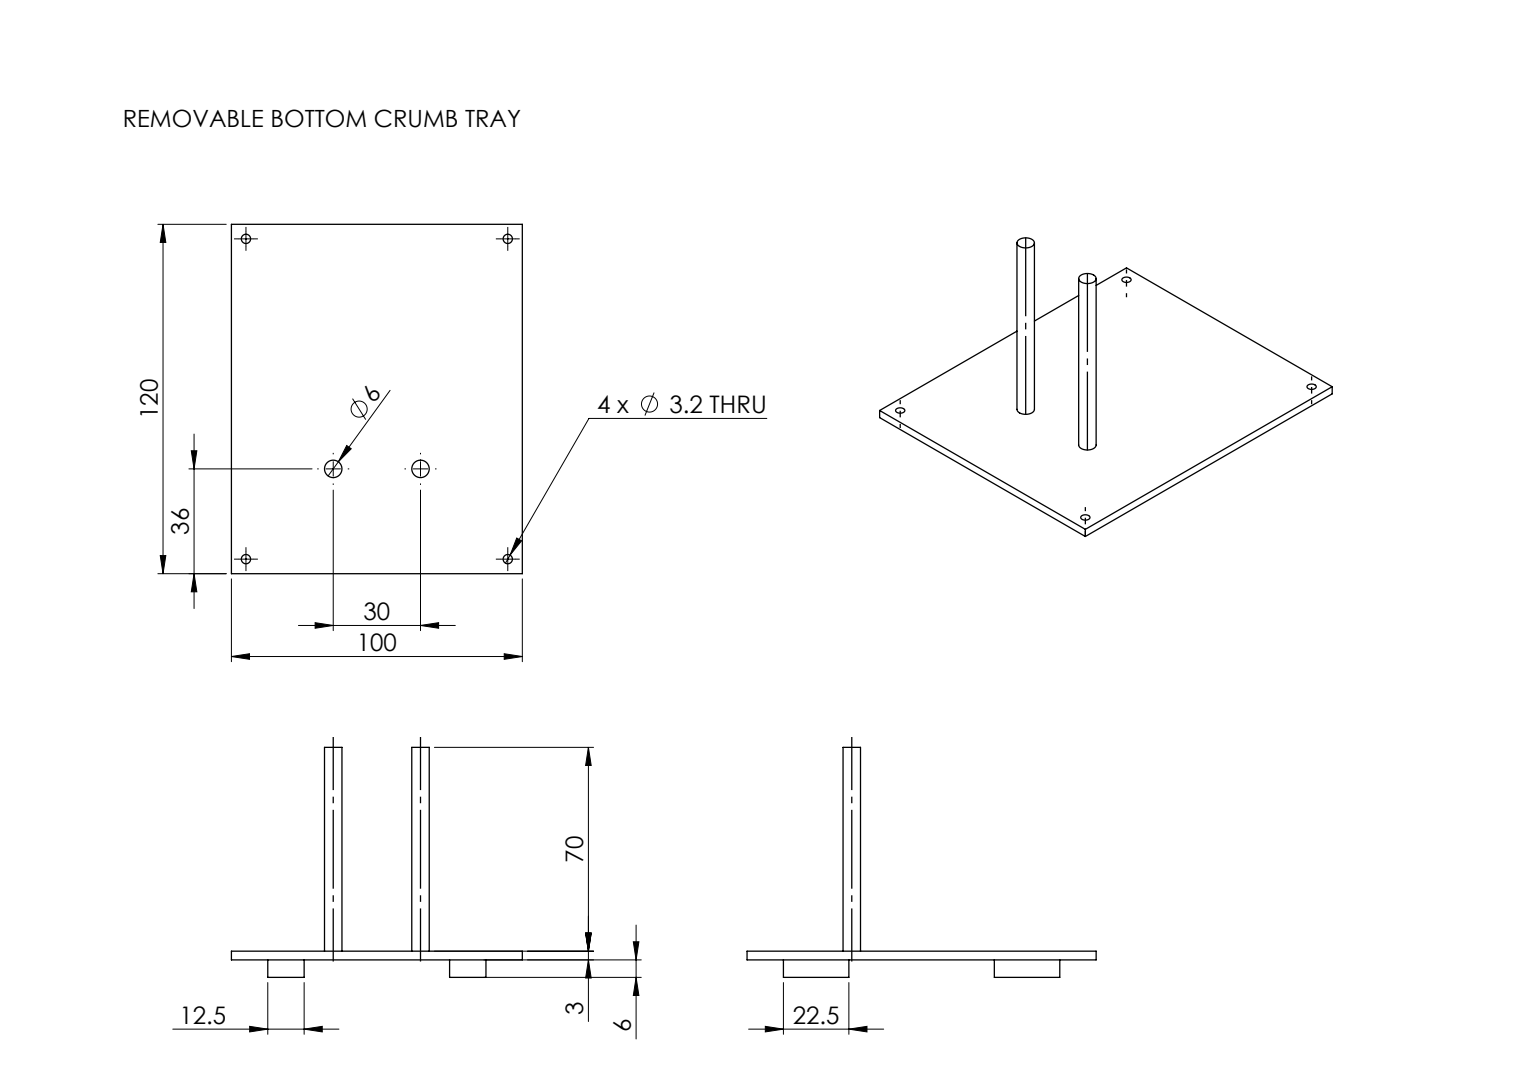
ISO-10303-21;
HEADER;
FILE_DESCRIPTION (('STEP AP214'),
    '1' );
FILE_NAME ('Removable Bottom Crumb Tray.step',
    '2026-10-08T14:41:38',
    ( '' ),
    ( '' ),
    'SwSTEP 2.0',
    'SolidWorks 2026',
    '' );
FILE_SCHEMA (( 'AUTOMOTIVE_DESIGN' ));
ENDSEC;

DATA;
#10=FACE_OUTER_BOUND ( 'NONE', #5278, .T. ) ;
#18=EDGE_CURVE ( 'NONE', #5079, #4517, #16249, .T. ) ;
#22=VECTOR ( 'NONE', #16690, 1000.000000000000000 ) ;
#26=EDGE_CURVE ( 'NONE', #14106, #19091, #11969, .T. ) ;
#36=EDGE_CURVE ( 'NONE', #18345, #7828, #11830, .T. ) ;
#43=CARTESIAN_POINT ( 'NONE',  ( 37.50000000000000711, -6.000000000000000000, -45.00000000000000000 ) ) ;
#62=CARTESIAN_POINT ( 'NONE',  ( -37.50000000000002132, 0.000000000000000000, 44.99999999999997868 ) ) ;
#75=FACE_OUTER_BOUND ( 'NONE', #12049, .T. ) ;
#86=LINE ( 'NONE', #12030, #9433 ) ;
#109=VERTEX_POINT ( 'NONE', #11046 ) ;
#116=CARTESIAN_POINT ( 'NONE',  ( -44.99999999999998579, 0.000000000000000000, -55.00000000000000000 ) ) ;
#124=EDGE_CURVE ( 'NONE', #10346, #18340, #3322, .T. ) ;
#138=EDGE_CURVE ( 'NONE', #19239, #1798, #9382, .T. ) ;
#157=DIRECTION ( 'NONE',  ( 1.000000000000000000, 0.000000000000000000, -7.709882115452476934E-17 ) ) ;
#163=LINE ( 'NONE', #1934, #7064 ) ;
#172=DIRECTION ( 'NONE',  ( -2.973811673103096679E-16, 0.000000000000000000, 1.000000000000000000 ) ) ;
#197=EDGE_LOOP ( 'NONE', ( #16436, #17465, #12376, #16579 ) ) ;
#223=LINE ( 'NONE', #13638, #15855 ) ;
#252=LINE ( 'NONE', #16158, #15418 ) ;
#255=DIRECTION ( 'NONE',  ( 0.000000000000000000, 0.000000000000000000, -1.000000000000000000 ) ) ;
#273=AXIS2_PLACEMENT_3D ( 'NONE', #16902, #3471, #9445 ) ;
#276=EDGE_CURVE ( 'NONE', #17921, #11844, #16850, .T. ) ;
#284=CARTESIAN_POINT ( 'NONE',  ( 14.99999999999998579, 3.000000000000000000, 26.99999999999997158 ) ) ;
#303=EDGE_CURVE ( 'NONE', #628, #8146, #5681, .T. ) ;
#315=LINE ( 'NONE', #7965, #7095 ) ;
#320=ORIENTED_EDGE ( 'NONE', *, *, #11499, .F. ) ;
#366=VECTOR ( 'NONE', #8391, 1000.000000000000000 ) ;
#370=LINE ( 'NONE', #15368, #6453 ) ;
#372=VECTOR ( 'NONE', #7310, 1000.000000000000000 ) ;
#378=ADVANCED_FACE ( 'NONE', ( #14562 ), #11224, .T. ) ;
#384=EDGE_CURVE ( 'NONE', #16449, #5562, #9851, .T. ) ;
#393=VECTOR ( 'NONE', #11200, 1000.000000000000000 ) ;
#394=EDGE_LOOP ( 'NONE', ( #6539, #4312, #7875, #13610 ) ) ;
#404=ORIENTED_EDGE ( 'NONE', *, *, #14193, .T. ) ;
#407=DIRECTION ( 'NONE',  ( -0.000000000000000000, -1.000000000000000000, -0.000000000000000000 ) ) ;
#423=EDGE_CURVE ( 'NONE', #13623, #11742, #14277, .T. ) ;
#428=VERTEX_POINT ( 'NONE', #16040 ) ;
#479=DIRECTION ( 'NONE',  ( -0.000000000000000000, -1.000000000000000000, -0.000000000000000000 ) ) ;
#497=DIRECTION ( 'NONE',  ( -1.000000000000000000, 0.000000000000000000, -9.251858538542970348E-17 ) ) ;
#510=EDGE_CURVE ( 'NONE', #15185, #7828, #9171, .T. ) ;
#526=EDGE_CURVE ( 'NONE', #18598, #13355, #19142, .T. ) ;
#528=EDGE_CURVE ( 'NONE', #3513, #14696, #14857, .T. ) ;
#539=DIRECTION ( 'NONE',  ( 0.000000000000000000, 0.000000000000000000, -1.000000000000000000 ) ) ;
#547=DIRECTION ( 'NONE',  ( 0.000000000000000000, 0.000000000000000000, -1.000000000000000000 ) ) ;
#553=ORIENTED_EDGE ( 'NONE', *, *, #12530, .T. ) ;
#561=EDGE_LOOP ( 'NONE', ( #1541, #12212 ) ) ;
#569=EDGE_CURVE ( 'NONE', #5562, #14997, #2796, .T. ) ;
#571=ADVANCED_BREP_SHAPE_REPRESENTATION ( '', ( #16938, #1791 ), #5851 ) ;
#572=DIRECTION ( 'NONE',  ( -1.541976423090495633E-16, 0.000000000000000000, 1.000000000000000000 ) ) ;
#577=ORIENTED_EDGE ( 'NONE', *, *, #17798, .T. ) ;
#589=EDGE_LOOP ( 'NONE', ( #3897, #9508, #16057, #4812 ) ) ;
#590=CARTESIAN_POINT ( 'NONE',  ( 44.99999999999998579, 0.000000000000000000, -54.99999999999998579 ) ) ;
#600=CARTESIAN_POINT ( 'NONE',  ( 44.99999999999998579, 3.000000000000000000, -53.39999999999999147 ) ) ;
#616=EDGE_CURVE ( 'NONE', #16789, #4517, #9072, .T. ) ;
#619=FACE_BOUND ( 'NONE', #18932, .T. ) ;
#628=VERTEX_POINT ( 'NONE', #13272 ) ;
#639=FACE_OUTER_BOUND ( 'NONE', #6765, .T. ) ;
#648=DIRECTION ( 'NONE',  ( -0.000000000000000000, -1.000000000000000000, -0.000000000000000000 ) ) ;
#654=EDGE_CURVE ( 'NONE', #10863, #8734, #2898, .T. ) ;
#673=PLANE ( 'NONE',  #15685 ) ;
#686=FACE_BOUND ( 'NONE', #17329, .T. ) ;
#717=VERTEX_POINT ( 'NONE', #15447 ) ;
#739=DIRECTION ( 'NONE',  ( 0.000000000000000000, -1.000000000000000000, 0.000000000000000000 ) ) ;
#762=EDGE_LOOP ( 'NONE', ( #16079, #7445, #9963, #6983 ) ) ;
#785=ADVANCED_FACE ( 'NONE', ( #639 ), #6236, .F. ) ;
#795=DIRECTION ( 'NONE',  ( -0.000000000000000000, -1.000000000000000000, -0.000000000000000000 ) ) ;
#821=EDGE_CURVE ( 'NONE', #5173, #12630, #4675, .T. ) ;
#830=CARTESIAN_POINT ( 'NONE',  ( -50.00000000000002132, 0.000000000000000000, -60.00000000000002132 ) ) ;
#848=EDGE_CURVE ( 'NONE', #5969, #14590, #7908, .T. ) ;
#865=ORIENTED_EDGE ( 'NONE', *, *, #15879, .F. ) ;
#887=EDGE_CURVE ( 'NONE', #16466, #19197, #4055, .T. ) ;
#894=DIRECTION ( 'NONE',  ( 0.000000000000000000, 0.000000000000000000, -1.000000000000000000 ) ) ;
#904=VECTOR ( 'NONE', #4505, 1000.000000000000000 ) ;
#945=AXIS2_PLACEMENT_3D ( 'NONE', #1086, #16280, #1182 ) ;
#985=CARTESIAN_POINT ( 'NONE',  ( -32.50000000000002132, -6.000000000000000000, -42.50000000000001421 ) ) ;
#1005=DIRECTION ( 'NONE',  ( -0.000000000000000000, -1.000000000000000000, -0.000000000000000000 ) ) ;
#1066=DIRECTION ( 'NONE',  ( 7.304098846218135653E-17, 0.000000000000000000, -1.000000000000000000 ) ) ;
#1069=DIRECTION ( 'NONE',  ( 0.000000000000000000, 0.000000000000000000, -1.000000000000000000 ) ) ;
#1086=CARTESIAN_POINT ( 'NONE',  ( -14.99999999999999645, 73.00000000000001421, 23.99999999999997868 ) ) ;
#1087=CYLINDRICAL_SURFACE ( 'NONE', #17377, 1.599999999999997202 ) ;
#1119=FACE_OUTER_BOUND ( 'NONE', #12928, .T. ) ;
#1130=AXIS2_PLACEMENT_3D ( 'NONE', #7594, #13560, #10719 ) ;
#1134=DIRECTION ( 'NONE',  ( -7.304098846218135653E-17, 0.000000000000000000, 1.000000000000000000 ) ) ;
#1165=LINE ( 'NONE', #4210, #17235 ) ;
#1168=VERTEX_POINT ( 'NONE', #6026 ) ;
#1182=DIRECTION ( 'NONE',  ( 0.000000000000000000, 0.000000000000000000, -1.000000000000000000 ) ) ;
#1183=PLANE ( 'NONE',  #5177 ) ;
#1225=EDGE_CURVE ( 'NONE', #5958, #13683, #9360, .T. ) ;
#1240=ORIENTED_EDGE ( 'NONE', *, *, #5077, .T. ) ;
#1242=EDGE_CURVE ( 'NONE', #3513, #7725, #3725, .T. ) ;
#1272=ORIENTED_EDGE ( 'NONE', *, *, #5680, .F. ) ;
#1298=AXIS2_PLACEMENT_3D ( 'NONE', #590, #15497, #8149 ) ;
#1302=AXIS2_PLACEMENT_3D ( 'NONE', #9765, #12794, #1134 ) ;
#1322=PLANE ( 'NONE',  #17661 ) ;
#1324=DIRECTION ( 'NONE',  ( 0.000000000000000000, 0.000000000000000000, -1.000000000000000000 ) ) ;
#1338=LINE ( 'NONE', #12006, #372 ) ;
#1344=ORIENTED_EDGE ( 'NONE', *, *, #13679, .F. ) ;
#1359=CARTESIAN_POINT ( 'NONE',  ( 37.49999999999999289, -6.000000000000000000, 47.49999999999997868 ) ) ;
#1374=CARTESIAN_POINT ( 'NONE',  ( 44.99999999999997158, -1.285879139104706187E-16, 55.00000000000000000 ) ) ;
#1379=CARTESIAN_POINT ( 'NONE',  ( -32.50000000000001421, -6.000000000000000000, 42.49999999999997868 ) ) ;
#1410=LINE ( 'NONE', #4162, #6882 ) ;
#1433=CIRCLE ( 'NONE', #3934, 1.599999999999997202 ) ;
#1434=LINE ( 'NONE', #17909, #15933 ) ;
#1469=EDGE_CURVE ( 'NONE', #16449, #6389, #7140, .T. ) ;
#1472=ORIENTED_EDGE ( 'NONE', *, *, #6683, .T. ) ;
#1473=ORIENTED_EDGE ( 'NONE', *, *, #18638, .T. ) ;
#1487=CARTESIAN_POINT ( 'NONE',  ( -37.50000000000002132, 107.3545527679194436, -25.00000000000002132 ) ) ;
#1501=ORIENTED_EDGE ( 'NONE', *, *, #15636, .T. ) ;
#1541=ORIENTED_EDGE ( 'NONE', *, *, #1225, .T. ) ;
#1550=VECTOR ( 'NONE', #9672, 1000.000000000000000 ) ;
#1556=ORIENTED_EDGE ( 'NONE', *, *, #2054, .F. ) ;
#1557=ORIENTED_EDGE ( 'NONE', *, *, #5324, .T. ) ;
#1565=PLANE ( 'NONE',  #2988 ) ;
#1567=ORIENTED_EDGE ( 'NONE', *, *, #5324, .F. ) ;
#1578=CARTESIAN_POINT ( 'NONE',  ( 44.99999999999997158, 3.000000000000000000, 53.40000000000000568 ) ) ;
#1579=PLANE ( 'NONE',  #7195 ) ;
#1596=EDGE_CURVE ( 'NONE', #8051, #6389, #5872, .T. ) ;
#1600=EDGE_LOOP ( 'NONE', ( #11359, #14227, #16909, #18115 ) ) ;
#1611=DIRECTION ( 'NONE',  ( -1.000000000000000000, 0.000000000000000000, 0.000000000000000000 ) ) ;
#1637=DIRECTION ( 'NONE',  ( -1.541976423090495880E-16, 0.000000000000000000, 1.000000000000000000 ) ) ;
#1670=ORIENTED_EDGE ( 'NONE', *, *, #15477, .T. ) ;
#1686=DIRECTION ( 'NONE',  ( -0.000000000000000000, 0.000000000000000000, -1.000000000000000000 ) ) ;
#1697=ORIENTED_EDGE ( 'NONE', *, *, #7811, .T. ) ;
#1699=EDGE_LOOP ( 'NONE', ( #18322, #18327, #18029, #18458 ) ) ;
#1729=CARTESIAN_POINT ( 'NONE',  ( 14.99999999999998579, 73.00000000000001421, 23.99999999999997158 ) ) ;
#1749=ORIENTED_EDGE ( 'NONE', *, *, #8582, .T. ) ;
#1750=ADVANCED_FACE ( 'NONE', ( #4605 ), #13604, .T. ) ;
#1753=ORIENTED_EDGE ( 'NONE', *, *, #9630, .F. ) ;
#1760=LINE ( 'NONE', #6371, #17711 ) ;
#1766=( NAMED_UNIT ( * ) PLANE_ANGLE_UNIT ( ) SI_UNIT ( $, .RADIAN. ) );
#1775=VECTOR ( 'NONE', #7172, 1000.000000000000000 ) ;
#1776=FACE_OUTER_BOUND ( 'NONE', #7352, .T. ) ;
#1777=ORIENTED_EDGE ( 'NONE', *, *, #12853, .F. ) ;
#1788=CARTESIAN_POINT ( 'NONE',  ( -37.50000000000002132, -6.000000000000000000, 47.49999999999997868 ) ) ;
#1791=AXIS2_PLACEMENT_3D ( 'NONE', #13713, #4815, #7646 ) ;
#1798=VERTEX_POINT ( 'NONE', #15472 ) ;
#1811=EDGE_CURVE ( 'NONE', #10346, #18257, #10858, .T. ) ;
#1831=CIRCLE ( 'NONE', #3394, 1.599999999999997202 ) ;
#1848=DIRECTION ( 'NONE',  ( -0.000000000000000000, -1.000000000000000000, -0.000000000000000000 ) ) ;
#1858=ORIENTED_EDGE ( 'NONE', *, *, #3600, .F. ) ;
#1859=EDGE_CURVE ( 'NONE', #18257, #10184, #2041, .T. ) ;
#1862=( NAMED_UNIT ( * ) SI_UNIT ( $, .STERADIAN. ) SOLID_ANGLE_UNIT ( ) );
#1895=AXIS2_PLACEMENT_3D ( 'NONE', #17069, #13828, #6484 ) ;
#1903=ADVANCED_FACE ( 'NONE', ( #15663 ), #8032, .T. ) ;
#1914=CIRCLE ( 'NONE', #12851, 1.599999999999997202 ) ;
#1921=EDGE_CURVE ( 'NONE', #2736, #14967, #6558, .T. ) ;
#1927=AXIS2_PLACEMENT_3D ( 'NONE', #19199, #10259, #10364 ) ;
#1934=CARTESIAN_POINT ( 'NONE',  ( 24.99999999999998579, 0.000000000000000000, 47.49999999999997868 ) ) ;
#1967=CARTESIAN_POINT ( 'NONE',  ( -35.00000000000002132, -0.000000000000000000, -42.50000000000001421 ) ) ;
#1971=DIRECTION ( 'NONE',  ( 0.000000000000000000, 1.000000000000000000, 0.000000000000000000 ) ) ;
#2025=ORIENTED_EDGE ( 'NONE', *, *, #8424, .T. ) ;
#2039=VECTOR ( 'NONE', #16607, 1000.000000000000000 ) ;
#2041=LINE ( 'NONE', #17136, #1550 ) ;
#2042=DIRECTION ( 'NONE',  ( -1.000000000000000000, 0.000000000000000000, -9.251858538542970348E-17 ) ) ;
#2050=VERTEX_POINT ( 'NONE', #2703 ) ;
#2054=EDGE_CURVE ( 'NONE', #19239, #2533, #5370, .T. ) ;
#2077=DIRECTION ( 'NONE',  ( -0.000000000000000000, -1.000000000000000000, -0.000000000000000000 ) ) ;
#2087=AXIS2_PLACEMENT_3D ( 'NONE', #7003, #18970, #1324 ) ;
#2104=FACE_OUTER_BOUND ( 'NONE', #8312, .T. ) ;
#2116=EDGE_CURVE ( 'NONE', #10863, #4229, #17606, .T. ) ;
#2147=ORIENTED_EDGE ( 'NONE', *, *, #3502, .F. ) ;
#2173=EDGE_LOOP ( 'NONE', ( #14107, #11827, #15804, #3822 ) ) ;
#2192=UNCERTAINTY_MEASURE_WITH_UNIT (LENGTH_MEASURE( 1.000000000000000082E-05 ), #3374, 'distance_accuracy_value', 'NONE');
#2230=DIRECTION ( 'NONE',  ( -0.000000000000000000, -1.000000000000000000, -0.000000000000000000 ) ) ;
#2233=DIRECTION ( 'NONE',  ( 0.000000000000000000, 1.000000000000000000, 0.000000000000000000 ) ) ;
#2237=VECTOR ( 'NONE', #15155, 1000.000000000000000 ) ;
#2272=FACE_OUTER_BOUND ( 'NONE', #762, .T. ) ;
#2273=ORIENTED_EDGE ( 'NONE', *, *, #12227, .T. ) ;
#2298=CARTESIAN_POINT ( 'NONE',  ( -25.00000000000001421, -6.000000000000000000, 47.49999999999997868 ) ) ;
#2310=ADVANCED_FACE ( 'NONE', ( #15062 ), #7612, .T. ) ;
#2317=ORIENTED_EDGE ( 'NONE', *, *, #4372, .F. ) ;
#2327=EDGE_CURVE ( 'NONE', #16010, #5207, #1831, .T. ) ;
#2333=ORIENTED_EDGE ( 'NONE', *, *, #18, .T. ) ;
#2350=DIRECTION ( 'NONE',  ( 0.000000000000000000, -1.000000000000000000, 0.000000000000000000 ) ) ;
#2369=ORIENTED_EDGE ( 'NONE', *, *, #7308, .F. ) ;
#2409=DIRECTION ( 'NONE',  ( -0.000000000000000000, -1.000000000000000000, -0.000000000000000000 ) ) ;
#2415=CARTESIAN_POINT ( 'NONE',  ( -35.00000000000002132, -6.000000000000000000, -47.50000000000002132 ) ) ;
#2416=VERTEX_POINT ( 'NONE', #7805 ) ;
#2437=FACE_OUTER_BOUND ( 'NONE', #11871, .T. ) ;
#2454=ORIENTED_EDGE ( 'NONE', *, *, #2913, .F. ) ;
#2461=CARTESIAN_POINT ( 'NONE',  ( 34.99999999999999289, -6.000000000000000000, 42.49999999999997868 ) ) ;
#2491=ORIENTED_EDGE ( 'NONE', *, *, #26, .T. ) ;
#2509=AXIS2_PLACEMENT_3D ( 'NONE', #6095, #15302, #12353 ) ;
#2520=VERTEX_POINT ( 'NONE', #830 ) ;
#2533=VERTEX_POINT ( 'NONE', #6812 ) ;
#2543=EDGE_LOOP ( 'NONE', ( #1272, #8187, #18133, #10701 ) ) ;
#2557=AXIS2_PLACEMENT_3D ( 'NONE', #116, #7461, #13432 ) ;
#2560=FACE_OUTER_BOUND ( 'NONE', #13945, .T. ) ;
#2561=FACE_OUTER_BOUND ( 'NONE', #8300, .T. ) ;
#2577=ORIENTED_EDGE ( 'NONE', *, *, #528, .T. ) ;
#2595=DIRECTION ( 'NONE',  ( -0.000000000000000000, -1.000000000000000000, -0.000000000000000000 ) ) ;
#2611=ORIENTED_EDGE ( 'NONE', *, *, #569, .F. ) ;
#2633=ADVANCED_FACE ( 'NONE', ( #619, #11006, #15527, #13754, #10714, #3373, #4762 ), #12184, .F. ) ;
#2643=ORIENTED_EDGE ( 'NONE', *, *, #848, .T. ) ;
#2684=VECTOR ( 'NONE', #17099, 1000.000000000000000 ) ;
#2703=CARTESIAN_POINT ( 'NONE',  ( -37.50000000000002132, -6.000000000000000000, 47.49999999999997868 ) ) ;
#2723=ADVANCED_FACE ( 'NONE', ( #16272 ), #1579, .F. ) ;
#2724=EDGE_LOOP ( 'NONE', ( #13146, #2369 ) ) ;
#2726=CARTESIAN_POINT ( 'NONE',  ( -32.50000000000001421, -6.000000000000000000, 24.99999999999998224 ) ) ;
#2736=VERTEX_POINT ( 'NONE', #1379 ) ;
#2752=CARTESIAN_POINT ( 'NONE',  ( -25.00000000000001421, -6.000000000000000000, 47.49999999999997868 ) ) ;
#2768=ORIENTED_EDGE ( 'NONE', *, *, #18009, .F. ) ;
#2796=LINE ( 'NONE', #7209, #15707 ) ;
#2801=VECTOR ( 'NONE', #7551, 1000.000000000000000 ) ;
#2820=ORIENTED_EDGE ( 'NONE', *, *, #36, .F. ) ;
#2840=ORIENTED_EDGE ( 'NONE', *, *, #138, .F. ) ;
#2845=VERTEX_POINT ( 'NONE', #15204 ) ;
#2860=EDGE_CURVE ( 'NONE', #5958, #717, #4624, .T. ) ;
#2875=CARTESIAN_POINT ( 'NONE',  ( 37.50000000000000711, -6.000000000000000000, -47.50000000000000000 ) ) ;
#2898=LINE ( 'NONE', #19369, #6240 ) ;
#2908=VERTEX_POINT ( 'NONE', #9689 ) ;
#2913=EDGE_CURVE ( 'NONE', #16200, #15859, #6576, .T. ) ;
#2923=ORIENTED_EDGE ( 'NONE', *, *, #26, .F. ) ;
#2942=ORIENTED_EDGE ( 'NONE', *, *, #5989, .T. ) ;
#2946=FACE_OUTER_BOUND ( 'NONE', #11157, .T. ) ;
#2949=LINE ( 'NONE', #11665, #3785 ) ;
#2969=CARTESIAN_POINT ( 'NONE',  ( 14.99999999999998579, 73.00000000000001421, 20.99999999999997513 ) ) ;
#2988=AXIS2_PLACEMENT_3D ( 'NONE', #17735, #16463, #11739 ) ;
#3005=VECTOR ( 'NONE', #8364, 1000.000000000000000 ) ;
#3021=CARTESIAN_POINT ( 'NONE',  ( -32.50000000000001421, 0.000000000000000000, 44.99999999999997868 ) ) ;
#3024=VECTOR ( 'NONE', #18924, 1000.000000000000000 ) ;
#3033=DIRECTION ( 'NONE',  ( 0.000000000000000000, 0.000000000000000000, -1.000000000000000000 ) ) ;
#3051=DIRECTION ( 'NONE',  ( 1.156482317317871725E-16, 0.000000000000000000, -1.000000000000000000 ) ) ;
#3052=PRODUCT_CONTEXT ( 'NONE', #7058, 'mechanical' ) ;
#3111=AXIS2_PLACEMENT_3D ( 'NONE', #14326, #14514, #894 ) ;
#3121=DIRECTION ( 'NONE',  ( 0.000000000000000000, -0.000000000000000000, -1.000000000000000000 ) ) ;
#3206=DIRECTION ( 'NONE',  ( 1.000000000000000000, 0.000000000000000000, 2.973811673103096679E-16 ) ) ;
#3213=ORIENTED_EDGE ( 'NONE', *, *, #11832, .T. ) ;
#3222=CARTESIAN_POINT ( 'NONE',  ( -37.50000000000002842, -0.000000000000000000, -47.50000000000002132 ) ) ;
#3226=CARTESIAN_POINT ( 'NONE',  ( 0.000000000000000000, -6.000000000000000000, 0.000000000000000000 ) ) ;
#3234=DIRECTION ( 'NONE',  ( 0.000000000000000000, 0.000000000000000000, 1.000000000000000000 ) ) ;
#3253=FACE_OUTER_BOUND ( 'NONE', #16379, .T. ) ;
#3269=ORIENTED_EDGE ( 'NONE', *, *, #384, .T. ) ;
#3272=CARTESIAN_POINT ( 'NONE',  ( 24.99999999999999289, -6.000000000000000000, -47.50000000000002132 ) ) ;
#3274=LINE ( 'NONE', #15136, #13277 ) ;
#3322=LINE ( 'NONE', #18424, #6036 ) ;
#3346=PLANE ( 'NONE',  #10336 ) ;
#3348=AXIS2_PLACEMENT_3D ( 'NONE', #18480, #3566, #5714 ) ;
#3350=ORIENTED_EDGE ( 'NONE', *, *, #13689, .T. ) ;
#3373=FACE_BOUND ( 'NONE', #5404, .T. ) ;
#3374=( LENGTH_UNIT ( ) NAMED_UNIT ( * ) SI_UNIT ( .MILLI., .METRE. ) );
#3375=CARTESIAN_POINT ( 'NONE',  ( 32.50000000000000000, 0.000000000000000000, -25.00000000000001421 ) ) ;
#3383=CARTESIAN_POINT ( 'NONE',  ( 24.99999999999998579, -6.000000000000000000, 47.49999999999997868 ) ) ;
#3387=CARTESIAN_POINT ( 'NONE',  ( 44.99999999999998579, -1.285879139104706187E-16, -54.99999999999998579 ) ) ;
#3393=CARTESIAN_POINT ( 'NONE',  ( 34.99999999999999289, 0.000000000000000000, 47.49999999999997868 ) ) ;
#3394=AXIS2_PLACEMENT_3D ( 'NONE', #16927, #17117, #547 ) ;
#3425=SHAPE_REPRESENTATION_RELATIONSHIP ( 'NONE' , 'NONE' ,  #13906, #571 ) ;
#3435=DIRECTION ( 'NONE',  ( 1.000000000000000000, 0.000000000000000000, -5.782411586589357392E-17 ) ) ;
#3440=DIRECTION ( 'NONE',  ( 0.000000000000000000, 0.000000000000000000, -1.000000000000000000 ) ) ;
#3455=VERTEX_POINT ( 'NONE', #16701 ) ;
#3471=DIRECTION ( 'NONE',  ( 0.000000000000000000, -1.000000000000000000, 0.000000000000000000 ) ) ;
#3477=VECTOR ( 'NONE', #12382, 1000.000000000000000 ) ;
#3482=CARTESIAN_POINT ( 'NONE',  ( 24.99999999999998579, 107.3545527679194436, 47.49999999999997868 ) ) ;
#3486=DIRECTION ( 'NONE',  ( -1.541976423090495880E-16, 0.000000000000000000, 1.000000000000000000 ) ) ;
#3502=EDGE_CURVE ( 'NONE', #5079, #1798, #16502, .T. ) ;
#3513=VERTEX_POINT ( 'NONE', #14833 ) ;
#3521=LINE ( 'NONE', #7841, #18197 ) ;
#3525=ORIENTED_EDGE ( 'NONE', *, *, #15477, .F. ) ;
#3566=DIRECTION ( 'NONE',  ( 0.000000000000000000, -1.000000000000000000, 0.000000000000000000 ) ) ;
#3567=CARTESIAN_POINT ( 'NONE',  ( -35.00000000000002132, -6.000000000000000000, -47.50000000000002132 ) ) ;
#3569=ORIENTED_EDGE ( 'NONE', *, *, #7811, .F. ) ;
#3598=ORIENTED_EDGE ( 'NONE', *, *, #3600, .T. ) ;
#3600=EDGE_CURVE ( 'NONE', #13252, #2050, #16998, .T. ) ;
#3606=CARTESIAN_POINT ( 'NONE',  ( -32.50000000000001421, -6.000000000000000000, 42.49999999999997868 ) ) ;
#3629=LINE ( 'NONE', #15401, #8186 ) ;
#3651=AXIS2_PLACEMENT_3D ( 'NONE', #7370, #16394, #4540 ) ;
#3665=CYLINDRICAL_SURFACE ( 'NONE', #5671, 1.599999999999997202 ) ;
#3677=DIRECTION ( 'NONE',  ( -0.000000000000000000, -1.000000000000000000, -0.000000000000000000 ) ) ;
#3725=LINE ( 'NONE', #10883, #17836 ) ;
#3730=VECTOR ( 'NONE', #3486, 1000.000000000000000 ) ;
#3753=CARTESIAN_POINT ( 'NONE',  ( 37.50000000000000711, -6.000000000000000000, -45.00000000000000000 ) ) ;
#3759=LINE ( 'NONE', #15725, #3005 ) ;
#3773=VECTOR ( 'NONE', #14128, 1000.000000000000000 ) ;
#3785=VECTOR ( 'NONE', #11964, 1000.000000000000000 ) ;
#3809=ORIENTED_EDGE ( 'NONE', *, *, #15473, .T. ) ;
#3811=EDGE_LOOP ( 'NONE', ( #4293, #15845, #8985, #10486, #15467, #15193 ) ) ;
#3818=ORIENTED_EDGE ( 'NONE', *, *, #7861, .F. ) ;
#3822=ORIENTED_EDGE ( 'NONE', *, *, #18, .F. ) ;
#3824=PLANE ( 'NONE',  #4039 ) ;
#3828=FACE_OUTER_BOUND ( 'NONE', #197, .T. ) ;
#3836=ORIENTED_EDGE ( 'NONE', *, *, #4490, .T. ) ;
#3856=ORIENTED_EDGE ( 'NONE', *, *, #8335, .F. ) ;
#3890=PLANE ( 'NONE',  #9263 ) ;
#3897=ORIENTED_EDGE ( 'NONE', *, *, #15636, .F. ) ;
#3934=AXIS2_PLACEMENT_3D ( 'NONE', #16068, #17443, #1069 ) ;
#3936=PRODUCT_DEFINITION_SHAPE ( 'NONE', 'NONE',  #15783 ) ;
#3945=FACE_OUTER_BOUND ( 'NONE', #11031, .T. ) ;
#3982=CARTESIAN_POINT ( 'NONE',  ( 37.50000000000000711, -6.000000000000000000, -47.50000000000000000 ) ) ;
#3986=ADVANCED_FACE ( 'NONE', ( #1776 ), #3346, .F. ) ;
#3995=ORIENTED_EDGE ( 'NONE', *, *, #2327, .T. ) ;
#4008=FACE_OUTER_BOUND ( 'NONE', #10455, .T. ) ;
#4011=EDGE_CURVE ( 'NONE', #14588, #16872, #3629, .T. ) ;
#4031=CARTESIAN_POINT ( 'NONE',  ( -37.50000000000002132, 0.000000000000000000, -25.00000000000002132 ) ) ;
#4039=AXIS2_PLACEMENT_3D ( 'NONE', #7139, #12823, #15691 ) ;
#4044=AXIS2_PLACEMENT_3D ( 'NONE', #3226, #16554, #3121 ) ;
#4052=LINE ( 'NONE', #8468, #9839 ) ;
#4054=CARTESIAN_POINT ( 'NONE',  ( -32.50000000000001421, -6.000000000000000000, 24.99999999999998224 ) ) ;
#4055=LINE ( 'NONE', #5531, #7792 ) ;
#4067=CIRCLE ( 'NONE', #17529, 1.599999999999997202 ) ;
#4089=ORIENTED_EDGE ( 'NONE', *, *, #11323, .T. ) ;
#4136=ORIENTED_EDGE ( 'NONE', *, *, #8424, .F. ) ;
#4137=LINE ( 'NONE', #5231, #15040 ) ;
#4162=CARTESIAN_POINT ( 'NONE',  ( -35.00000000000002132, -0.000000000000000000, -47.50000000000002132 ) ) ;
#4183=DIRECTION ( 'NONE',  ( -1.000000000000000000, -0.000000000000000000, -2.081668171172167774E-16 ) ) ;
#4200=EDGE_LOOP ( 'NONE', ( #10665, #7038 ) ) ;
#4201=LINE ( 'NONE', #2726, #18205 ) ;
#4205=CARTESIAN_POINT ( 'NONE',  ( 24.99999999999998579, 0.000000000000000000, 42.49999999999997868 ) ) ;
#4210=CARTESIAN_POINT ( 'NONE',  ( -50.00000000000001421, 3.000000000000000000, 59.99999999999997868 ) ) ;
#4219=CIRCLE ( 'NONE', #12364, 1.599999999999997202 ) ;
#4223=FACE_OUTER_BOUND ( 'NONE', #6540, .T. ) ;
#4228=DIRECTION ( 'NONE',  ( 0.000000000000000000, 0.000000000000000000, -1.000000000000000000 ) ) ;
#4229=VERTEX_POINT ( 'NONE', #11160 ) ;
#4231=DIRECTION ( 'NONE',  ( 0.000000000000000000, -1.000000000000000000, 0.000000000000000000 ) ) ;
#4242=DIRECTION ( 'NONE',  ( -1.000000000000000000, 0.000000000000000000, -9.251858538542970348E-17 ) ) ;
#4258=EDGE_CURVE ( 'NONE', #4857, #9993, #4201, .T. ) ;
#4262=ADVANCED_FACE ( 'NONE', ( #5767 ), #8697, .F. ) ;
#4280=LINE ( 'NONE', #16226, #9663 ) ;
#4290=ORIENTED_EDGE ( 'NONE', *, *, #10424, .F. ) ;
#4293=ORIENTED_EDGE ( 'NONE', *, *, #4849, .F. ) ;
#4299=ORIENTED_EDGE ( 'NONE', *, *, #2116, .T. ) ;
#4310=DIRECTION ( 'NONE',  ( -1.000000000000000000, 0.000000000000000000, 0.000000000000000000 ) ) ;
#4312=ORIENTED_EDGE ( 'NONE', *, *, #5196, .F. ) ;
#4350=DIRECTION ( 'NONE',  ( -1.000000000000000000, 0.000000000000000000, 0.000000000000000000 ) ) ;
#4354=EDGE_CURVE ( 'NONE', #17877, #428, #6918, .T. ) ;
#4372=EDGE_CURVE ( 'NONE', #11522, #6502, #86, .T. ) ;
#4377=DIRECTION ( 'NONE',  ( -0.000000000000000000, -1.000000000000000000, -0.000000000000000000 ) ) ;
#4392=ORIENTED_EDGE ( 'NONE', *, *, #17824, .F. ) ;
#4410=AXIS2_PLACEMENT_3D ( 'NONE', #11939, #14681, #17826 ) ;
#4422=DIRECTION ( 'NONE',  ( -0.000000000000000000, -1.000000000000000000, -0.000000000000000000 ) ) ;
#4423=CARTESIAN_POINT ( 'NONE',  ( 44.99999999999997158, 0.000000000000000000, 53.40000000000000568 ) ) ;
#4434=CARTESIAN_POINT ( 'NONE',  ( 37.49999999999999289, 0.000000000000000000, 47.49999999999997868 ) ) ;
#4458=LINE ( 'NONE', #4759, #10788 ) ;
#4490=EDGE_CURVE ( 'NONE', #14696, #10900, #13994, .T. ) ;
#4493=ORIENTED_EDGE ( 'NONE', *, *, #1811, .T. ) ;
#4505=DIRECTION ( 'NONE',  ( 7.304098846218135653E-17, 0.000000000000000000, -1.000000000000000000 ) ) ;
#4514=ORIENTED_EDGE ( 'NONE', *, *, #12227, .F. ) ;
#4517=VERTEX_POINT ( 'NONE', #3222 ) ;
#4518=ORIENTED_EDGE ( 'NONE', *, *, #11514, .F. ) ;
#4540=DIRECTION ( 'NONE',  ( 0.000000000000000000, -0.000000000000000000, -1.000000000000000000 ) ) ;
#4551=PLANE ( 'NONE',  #8434 ) ;
#4552=LINE ( 'NONE', #7684, #2039 ) ;
#4555=DIRECTION ( 'NONE',  ( 0.000000000000000000, 0.000000000000000000, -1.000000000000000000 ) ) ;
#4563=ORIENTED_EDGE ( 'NONE', *, *, #15828, .T. ) ;
#4577=LINE ( 'NONE', #5746, #11537 ) ;
#4581=DIRECTION ( 'NONE',  ( 0.000000000000000000, 1.000000000000000000, 0.000000000000000000 ) ) ;
#4584=ORIENTED_EDGE ( 'NONE', *, *, #10831, .F. ) ;
#4605=FACE_OUTER_BOUND ( 'NONE', #8909, .T. ) ;
#4612=FACE_OUTER_BOUND ( 'NONE', #589, .T. ) ;
#4613=ORIENTED_EDGE ( 'NONE', *, *, #616, .F. ) ;
#4617=DIRECTION ( 'NONE',  ( 0.000000000000000000, 1.000000000000000000, 0.000000000000000000 ) ) ;
#4623=DIRECTION ( 'NONE',  ( 0.000000000000000000, 0.000000000000000000, -1.000000000000000000 ) ) ;
#4624=LINE ( 'NONE', #4423, #2801 ) ;
#4632=CARTESIAN_POINT ( 'NONE',  ( 44.99999999999998579, -1.285879139104706187E-16, -54.99999999999998579 ) ) ;
#4649=ORIENTED_EDGE ( 'NONE', *, *, #528, .F. ) ;
#4671=CARTESIAN_POINT ( 'NONE',  ( -45.00000000000000000, -1.285879139104706187E-16, 54.99999999999998579 ) ) ;
#4675=CIRCLE ( 'NONE', #17487, 1.599999999999997202 ) ;
#4679=CARTESIAN_POINT ( 'NONE',  ( 32.49999999999998579, -6.000000000000000000, -25.00000000000001421 ) ) ;
#4692=VECTOR ( 'NONE', #1848, 1000.000000000000000 ) ;
#4713=EDGE_LOOP ( 'NONE', ( #9586, #4299, #5794, #4493 ) ) ;
#4743=DIRECTION ( 'NONE',  ( 0.000000000000000000, -1.000000000000000000, 0.000000000000000000 ) ) ;
#4759=CARTESIAN_POINT ( 'NONE',  ( 37.50000000000000711, -6.000000000000000000, -45.00000000000000000 ) ) ;
#4762=FACE_OUTER_BOUND ( 'NONE', #4713, .T. ) ;
#4765=PRESENTATION_STYLE_ASSIGNMENT (( #6222 ) ) ;
#4812=ORIENTED_EDGE ( 'NONE', *, *, #569, .T. ) ;
#4815=DIRECTION ( 'NONE',  ( 0.000000000000000000, 0.000000000000000000, 1.000000000000000000 ) ) ;
#4817=ORIENTED_EDGE ( 'NONE', *, *, #11514, .T. ) ;
#4835=LINE ( 'NONE', #1788, #10812 ) ;
#4849=EDGE_CURVE ( 'NONE', #8051, #11742, #1410, .T. ) ;
#4857=VERTEX_POINT ( 'NONE', #4054 ) ;
#4901=LINE ( 'NONE', #17048, #12567 ) ;
#4924=CARTESIAN_POINT ( 'NONE',  ( -50.00000000000001421, 3.000000000000000000, 59.99999999999997868 ) ) ;
#5013=DIRECTION ( 'NONE',  ( -5.782411586589357392E-17, 0.000000000000000000, -1.000000000000000000 ) ) ;
#5014=ORIENTED_EDGE ( 'NONE', *, *, #15260, .T. ) ;
#5016=ORIENTED_EDGE ( 'NONE', *, *, #2860, .F. ) ;
#5018=DIRECTION ( 'NONE',  ( 0.000000000000000000, 0.000000000000000000, -1.000000000000000000 ) ) ;
#5077=EDGE_CURVE ( 'NONE', #5207, #16010, #4067, .T. ) ;
#5079=VERTEX_POINT ( 'NONE', #10977 ) ;
#5096=ADVANCED_FACE ( 'NONE', ( #4008 ), #3824, .T. ) ;
#5098=ADVANCED_FACE ( 'NONE', ( #2437 ), #5577, .T. ) ;
#5132=DIRECTION ( 'NONE',  ( -1.541976423090495880E-16, 0.000000000000000000, 1.000000000000000000 ) ) ;
#5173=VERTEX_POINT ( 'NONE', #17345 ) ;
#5174=PRODUCT_DEFINITION_FORMATION_WITH_SPECIFIED_SOURCE ( 'ANY', '', #12846, .NOT_KNOWN. ) ;
#5177=AXIS2_PLACEMENT_3D ( 'NONE', #17459, #8358, #7163 ) ;
#5196=EDGE_CURVE ( 'NONE', #18345, #11522, #9881, .T. ) ;
#5207=VERTEX_POINT ( 'NONE', #17438 ) ;
#5221=DIRECTION ( 'NONE',  ( 0.000000000000000000, -1.000000000000000000, 0.000000000000000000 ) ) ;
#5231=CARTESIAN_POINT ( 'NONE',  ( 34.99999999999999289, -6.000000000000000000, 42.49999999999997868 ) ) ;
#5237=AXIS2_PLACEMENT_3D ( 'NONE', #7255, #14995, #7545 ) ;
#5241=PLANE ( 'NONE',  #11753 ) ;
#5259=ORIENTED_EDGE ( 'NONE', *, *, #17753, .T. ) ;
#5270=CARTESIAN_POINT ( 'NONE',  ( -14.99999999999999645, 73.00000000000001421, 23.99999999999997868 ) ) ;
#5278=EDGE_LOOP ( 'NONE', ( #1697, #8501, #9253, #15208 ) ) ;
#5294=CARTESIAN_POINT ( 'NONE',  ( -35.00000000000002132, -6.000000000000000000, -42.50000000000001421 ) ) ;
#5307=DIRECTION ( 'NONE',  ( 0.000000000000000000, 0.000000000000000000, -1.000000000000000000 ) ) ;
#5318=ORIENTED_EDGE ( 'NONE', *, *, #12280, .F. ) ;
#5324=EDGE_CURVE ( 'NONE', #13252, #14588, #17728, .T. ) ;
#5368=EDGE_CURVE ( 'NONE', #14967, #9993, #11942, .T. ) ;
#5370=LINE ( 'NONE', #18794, #7462 ) ;
#5385=VECTOR ( 'NONE', #15271, 1000.000000000000000 ) ;
#5386=PLANE ( 'NONE',  #17911 ) ;
#5389=ORIENTED_EDGE ( 'NONE', *, *, #10675, .T. ) ;
#5400=VECTOR ( 'NONE', #16653, 1000.000000000000000 ) ;
#5404=EDGE_LOOP ( 'NONE', ( #3525, #11161 ) ) ;
#5406=LINE ( 'NONE', #985, #9277 ) ;
#5443=CARTESIAN_POINT ( 'NONE',  ( 44.99999999999997158, 0.000000000000000000, 55.00000000000000000 ) ) ;
#5449=CARTESIAN_POINT ( 'NONE',  ( 44.99999999999997158, 0.000000000000000000, 55.00000000000000000 ) ) ;
#5455=DIRECTION ( 'NONE',  ( -0.000000000000000000, 1.000000000000000000, -0.000000000000000000 ) ) ;
#5472=LINE ( 'NONE', #7033, #14456 ) ;
#5531=CARTESIAN_POINT ( 'NONE',  ( 37.49999999999999289, 107.3545527679194436, -25.00000000000001421 ) ) ;
#5546=CARTESIAN_POINT ( 'NONE',  ( 50.00000000000000000, 3.000000000000000000, -60.00000000000000000 ) ) ;
#5558=EDGE_LOOP ( 'NONE', ( #12166, #2577, #12505, #4584 ) ) ;
#5562=VERTEX_POINT ( 'NONE', #8677 ) ;
#5574=LINE ( 'NONE', #8329, #6886 ) ;
#5577=PLANE ( 'NONE',  #6853 ) ;
#5580=EDGE_CURVE ( 'NONE', #17240, #2533, #1434, .T. ) ;
#5599=ORIENTED_EDGE ( 'NONE', *, *, #19379, .F. ) ;
#5601=DIRECTION ( 'NONE',  ( -0.000000000000000000, -1.000000000000000000, -0.000000000000000000 ) ) ;
#5671=AXIS2_PLACEMENT_3D ( 'NONE', #14430, #1005, #14151 ) ;
#5680=EDGE_CURVE ( 'NONE', #13683, #2416, #4577, .T. ) ;
#5681=CIRCLE ( 'NONE', #8808, 1.599999999999997202 ) ;
#5697=EDGE_CURVE ( 'NONE', #9017, #17877, #4280, .T. ) ;
#5704=DIRECTION ( 'NONE',  ( 0.000000000000000000, -1.000000000000000000, 0.000000000000000000 ) ) ;
#5707=DIRECTION ( 'NONE',  ( 0.000000000000000000, 0.000000000000000000, -1.000000000000000000 ) ) ;
#5714=DIRECTION ( 'NONE',  ( 0.000000000000000000, 0.000000000000000000, -1.000000000000000000 ) ) ;
#5746=CARTESIAN_POINT ( 'NONE',  ( 44.99999999999997158, 0.000000000000000000, 56.59999999999999432 ) ) ;
#5767=FACE_OUTER_BOUND ( 'NONE', #7732, .T. ) ;
#5794=ORIENTED_EDGE ( 'NONE', *, *, #9280, .T. ) ;
#5851=( GEOMETRIC_REPRESENTATION_CONTEXT ( 3 ) GLOBAL_UNCERTAINTY_ASSIGNED_CONTEXT ( ( #14154 ) ) GLOBAL_UNIT_ASSIGNED_CONTEXT ( ( #15196, #1766, #6471 ) ) REPRESENTATION_CONTEXT ( 'NONE', 'WORKASPACE' ) );
#5862=DIRECTION ( 'NONE',  ( -1.541976423090495633E-16, 0.000000000000000000, 1.000000000000000000 ) ) ;
#5872=LINE ( 'NONE', #10562, #4692 ) ;
#5879=ADVANCED_FACE ( 'NONE', ( #17648 ), #16377, .T. ) ;
#5884=EDGE_LOOP ( 'NONE', ( #3569, #4514, #13419, #7979 ) ) ;
#5887=DIRECTION ( 'NONE',  ( -1.541976423090495880E-16, 0.000000000000000000, 1.000000000000000000 ) ) ;
#5888=DIRECTION ( 'NONE',  ( -2.081668171172167774E-16, 0.000000000000000000, 1.000000000000000000 ) ) ;
#5891=EDGE_CURVE ( 'NONE', #18739, #5079, #17948, .T. ) ;
#5898=CARTESIAN_POINT ( 'NONE',  ( -32.50000000000002132, 0.000000000000000000, -25.00000000000002842 ) ) ;
#5900=CYLINDRICAL_SURFACE ( 'NONE', #2557, 1.599999999999997202 ) ;
#5917=CARTESIAN_POINT ( 'NONE',  ( 44.99999999999997158, 3.000000000000000000, 56.59999999999999432 ) ) ;
#5934=DIRECTION ( 'NONE',  ( 1.156482317317871725E-16, 0.000000000000000000, -1.000000000000000000 ) ) ;
#5958=VERTEX_POINT ( 'NONE', #1578 ) ;
#5969=VERTEX_POINT ( 'NONE', #10479 ) ;
#5984=VECTOR ( 'NONE', #3051, 1000.000000000000000 ) ;
#5989=EDGE_CURVE ( 'NONE', #11742, #16466, #16472, .T. ) ;
#6001=DIRECTION ( 'NONE',  ( 7.304098846218135653E-17, 0.000000000000000000, -1.000000000000000000 ) ) ;
#6010=PLANE ( 'NONE',  #3651 ) ;
#6026=CARTESIAN_POINT ( 'NONE',  ( 37.49999999999999289, -6.000000000000000000, 24.99999999999998579 ) ) ;
#6036=VECTOR ( 'NONE', #9291, 1000.000000000000000 ) ;
#6039=ADVANCED_FACE ( 'NONE', ( #4223 ), #18440, .F. ) ;
#6092=ORIENTED_EDGE ( 'NONE', *, *, #18557, .F. ) ;
#6093=DIRECTION ( 'NONE',  ( -1.000000000000000000, 0.000000000000000000, -1.156482317317871725E-16 ) ) ;
#6095=CARTESIAN_POINT ( 'NONE',  ( -25.00000000000001421, 107.3545527679194436, 47.49999999999997868 ) ) ;
#6122=DIRECTION ( 'NONE',  ( 0.000000000000000000, -1.000000000000000000, 0.000000000000000000 ) ) ;
#6150=DIRECTION ( 'NONE',  ( -7.304098846218135653E-17, 0.000000000000000000, 1.000000000000000000 ) ) ;
#6173=VECTOR ( 'NONE', #10474, 1000.000000000000000 ) ;
#6176=AXIS2_PLACEMENT_3D ( 'NONE', #5443, #7098, #15924 ) ;
#6180=CARTESIAN_POINT ( 'NONE',  ( 37.49999999999999289, 107.3545527679194436, 24.99999999999998579 ) ) ;
#6184=EDGE_CURVE ( 'NONE', #8734, #2520, #17776, .T. ) ;
#6188=EDGE_LOOP ( 'NONE', ( #553, #2025 ) ) ;
#6202=DIRECTION ( 'NONE',  ( -1.541976423090495880E-16, 0.000000000000000000, 1.000000000000000000 ) ) ;
#6206=DIRECTION ( 'NONE',  ( -0.000000000000000000, 1.000000000000000000, -0.000000000000000000 ) ) ;
#6208=FACE_OUTER_BOUND ( 'NONE', #12180, .T. ) ;
#6215=LINE ( 'NONE', #19347, #9680 ) ;
#6222=SURFACE_STYLE_USAGE ( .BOTH. , #12387 ) ;
#6224=FACE_OUTER_BOUND ( 'NONE', #18804, .T. ) ;
#6236=CYLINDRICAL_SURFACE ( 'NONE', #9667, 1.599999999999997202 ) ;
#6240=VECTOR ( 'NONE', #11911, 1000.000000000000000 ) ;
#6269=AXIS2_PLACEMENT_3D ( 'NONE', #1487, #13232, #13425 ) ;
#6270=CARTESIAN_POINT ( 'NONE',  ( -37.50000000000002132, 107.3545527679194436, -25.00000000000002132 ) ) ;
#6280=ADVANCED_FACE ( 'NONE', ( #8946 ), #4551, .F. ) ;
#6298=DIRECTION ( 'NONE',  ( 5.782411586589357392E-17, -0.000000000000000000, 1.000000000000000000 ) ) ;
#6371=CARTESIAN_POINT ( 'NONE',  ( -14.99999999999999645, 73.00000000000001421, 26.99999999999997868 ) ) ;
#6387=ORIENTED_EDGE ( 'NONE', *, *, #7861, .T. ) ;
#6389=VERTEX_POINT ( 'NONE', #3272 ) ;
#6391=PLANE ( 'NONE',  #2509 ) ;
#6396=CARTESIAN_POINT ( 'NONE',  ( 24.99999999999999289, 0.000000000000000000, -42.50000000000001421 ) ) ;
#6409=CARTESIAN_POINT ( 'NONE',  ( 34.99999999999999289, -6.000000000000000000, 47.49999999999997868 ) ) ;
#6416=STYLED_ITEM ( 'NONE', ( #4765 ), #16938 ) ;
#6433=DIRECTION ( 'NONE',  ( 0.000000000000000000, 0.000000000000000000, -1.000000000000000000 ) ) ;
#6448=ORIENTED_EDGE ( 'NONE', *, *, #9630, .T. ) ;
#6453=VECTOR ( 'NONE', #7925, 1000.000000000000000 ) ;
#6461=DIRECTION ( 'NONE',  ( 0.000000000000000000, -0.000000000000000000, 1.000000000000000000 ) ) ;
#6471=( NAMED_UNIT ( * ) SI_UNIT ( $, .STERADIAN. ) SOLID_ANGLE_UNIT ( ) );
#6483=CIRCLE ( 'NONE', #3348, 1.599999999999997202 ) ;
#6484=DIRECTION ( 'NONE',  ( -7.709882115452476934E-17, 0.000000000000000000, -1.000000000000000000 ) ) ;
#6500=CIRCLE ( 'NONE', #16175, 2.999999999999999112 ) ;
#6502=VERTEX_POINT ( 'NONE', #14145 ) ;
#6509=ORIENTED_EDGE ( 'NONE', *, *, #5077, .F. ) ;
#6539=ORIENTED_EDGE ( 'NONE', *, *, #11499, .T. ) ;
#6540=EDGE_LOOP ( 'NONE', ( #16889, #7736, #10864, #16239 ) ) ;
#6558=LINE ( 'NONE', #3606, #10301 ) ;
#6566=CARTESIAN_POINT ( 'NONE',  ( -14.99999999999999645, 3.000000000000000000, 23.99999999999997868 ) ) ;
#6569=EDGE_LOOP ( 'NONE', ( #4392, #6761, #2820, #1344 ) ) ;
#6576=LINE ( 'NONE', #1967, #15031 ) ;
#6583=ORIENTED_EDGE ( 'NONE', *, *, #13319, .F. ) ;
#6622=ADVANCED_FACE ( 'NONE', ( #2560 ), #14516, .T. ) ;
#6650=VECTOR ( 'NONE', #14651, 1000.000000000000000 ) ;
#6661=ORIENTED_EDGE ( 'NONE', *, *, #3502, .T. ) ;
#6670=FACE_BOUND ( 'NONE', #16051, .T. ) ;
#6683=EDGE_CURVE ( 'NONE', #19310, #8146, #2949, .T. ) ;
#6709=COLOUR_RGB ( '', 0.40784314, 0.44705882, 0.49803922) ;
#6729=CARTESIAN_POINT ( 'NONE',  ( -32.50000000000002132, -6.000000000000000000, -42.50000000000001421 ) ) ;
#6742=ORIENTED_EDGE ( 'NONE', *, *, #17824, .T. ) ;
#6755=FACE_BOUND ( 'NONE', #3811, .T. ) ;
#6761=ORIENTED_EDGE ( 'NONE', *, *, #510, .T. ) ;
#6765=EDGE_LOOP ( 'NONE', ( #9879, #3809, #13940, #1777 ) ) ;
#6766=CARTESIAN_POINT ( 'NONE',  ( 32.49999999999998579, -6.000000000000000000, 24.99999999999998579 ) ) ;
#6780=CARTESIAN_POINT ( 'NONE',  ( -37.50000000000002132, -6.000000000000000000, 44.99999999999997868 ) ) ;
#6802=EDGE_CURVE ( 'NONE', #12630, #5173, #15377, .T. ) ;
#6812=CARTESIAN_POINT ( 'NONE',  ( -25.00000000000000711, 0.000000000000000000, -42.50000000000001421 ) ) ;
#6835=ORIENTED_EDGE ( 'NONE', *, *, #5580, .F. ) ;
#6853=AXIS2_PLACEMENT_3D ( 'NONE', #5294, #9791, #9969 ) ;
#6882=VECTOR ( 'NONE', #19351, 1000.000000000000000 ) ;
#6886=VECTOR ( 'NONE', #12917, 1000.000000000000000 ) ;
#6907=ADVANCED_FACE ( 'NONE', ( #15408 ), #6391, .F. ) ;
#6911=ORIENTED_EDGE ( 'NONE', *, *, #14804, .T. ) ;
#6918=CIRCLE ( 'NONE', #1927, 2.999999999999999112 ) ;
#6922=DIRECTION ( 'NONE',  ( 0.000000000000000000, 0.000000000000000000, -1.000000000000000000 ) ) ;
#6925=DIRECTION ( 'NONE',  ( -7.304098846218135653E-17, 0.000000000000000000, 1.000000000000000000 ) ) ;
#6961=DIRECTION ( 'NONE',  ( 0.000000000000000000, 0.000000000000000000, -1.000000000000000000 ) ) ;
#6970=ORIENTED_EDGE ( 'NONE', *, *, #15473, .F. ) ;
#6983=ORIENTED_EDGE ( 'NONE', *, *, #19379, .T. ) ;
#6990=ORIENTED_EDGE ( 'NONE', *, *, #8897, .F. ) ;
#6991=CARTESIAN_POINT ( 'NONE',  ( 37.50000000000000711, 0.000000000000000000, -47.50000000000000000 ) ) ;
#7003=CARTESIAN_POINT ( 'NONE',  ( 14.99999999999998579, 3.000000000000000000, 23.99999999999997158 ) ) ;
#7012=ADVANCED_FACE ( 'NONE', ( #75 ), #16146, .T. ) ;
#7033=CARTESIAN_POINT ( 'NONE',  ( -25.00000000000000711, -6.000000000000000000, -42.50000000000001421 ) ) ;
#7038=ORIENTED_EDGE ( 'NONE', *, *, #10033, .T. ) ;
#7058=APPLICATION_CONTEXT ( 'automotive_design' ) ;
#7064=VECTOR ( 'NONE', #6150, 1000.000000000000000 ) ;
#7090=CARTESIAN_POINT ( 'NONE',  ( -45.00000000000000000, -1.285879139104706187E-16, 56.59999999999998010 ) ) ;
#7095=VECTOR ( 'NONE', #6298, 1000.000000000000000 ) ;
#7098=DIRECTION ( 'NONE',  ( -0.000000000000000000, -1.000000000000000000, -0.000000000000000000 ) ) ;
#7134=DIRECTION ( 'NONE',  ( 0.000000000000000000, 1.000000000000000000, 0.000000000000000000 ) ) ;
#7139=CARTESIAN_POINT ( 'NONE',  ( -37.50000000000002132, 107.3545527679194436, 24.99999999999998224 ) ) ;
#7140=LINE ( 'NONE', #13107, #10615 ) ;
#7145=EDGE_CURVE ( 'NONE', #14590, #10761, #7785, .T. ) ;
#7163=DIRECTION ( 'NONE',  ( -1.541976423090495633E-16, 0.000000000000000000, 1.000000000000000000 ) ) ;
#7167=LINE ( 'NONE', #14170, #12267 ) ;
#7172=DIRECTION ( 'NONE',  ( 0.000000000000000000, 1.000000000000000000, 0.000000000000000000 ) ) ;
#7195=AXIS2_PLACEMENT_3D ( 'NONE', #16378, #5888, #8826 ) ;
#7209=CARTESIAN_POINT ( 'NONE',  ( 32.50000000000000000, -6.000000000000000000, -45.00000000000000000 ) ) ;
#7211=DIRECTION ( 'NONE',  ( -0.000000000000000000, -1.000000000000000000, -0.000000000000000000 ) ) ;
#7226=CARTESIAN_POINT ( 'NONE',  ( -35.00000000000002132, -6.000000000000000000, -42.50000000000001421 ) ) ;
#7238=ORIENTED_EDGE ( 'NONE', *, *, #887, .F. ) ;
#7239=CARTESIAN_POINT ( 'NONE',  ( 34.99999999999999289, -6.000000000000000000, 42.49999999999997868 ) ) ;
#7255=CARTESIAN_POINT ( 'NONE',  ( 0.000000000000000000, -6.000000000000000000, 0.000000000000000000 ) ) ;
#7270=AXIS2_PLACEMENT_3D ( 'NONE', #13868, #14061, #539 ) ;
#7308=EDGE_CURVE ( 'NONE', #13355, #18598, #1914, .T. ) ;
#7310=DIRECTION ( 'NONE',  ( -7.304098846218135653E-17, 0.000000000000000000, 1.000000000000000000 ) ) ;
#7324=FACE_OUTER_BOUND ( 'NONE', #7556, .T. ) ;
#7338=DIRECTION ( 'NONE',  ( 1.000000000000000000, 0.000000000000000000, 2.973811673103096679E-16 ) ) ;
#7350=EDGE_CURVE ( 'NONE', #13623, #19197, #12581, .T. ) ;
#7351=CARTESIAN_POINT ( 'NONE',  ( -37.50000000000002132, -6.000000000000000000, 44.99999999999997868 ) ) ;
#7352=EDGE_LOOP ( 'NONE', ( #18802, #11745, #13851, #16995 ) ) ;
#7364=AXIS2_PLACEMENT_3D ( 'NONE', #2461, #14424, #13035 ) ;
#7370=CARTESIAN_POINT ( 'NONE',  ( 0.000000000000000000, -6.000000000000000000, 0.000000000000000000 ) ) ;
#7429=ORIENTED_EDGE ( 'NONE', *, *, #276, .T. ) ;
#7445=ORIENTED_EDGE ( 'NONE', *, *, #19337, .F. ) ;
#7446=ORIENTED_EDGE ( 'NONE', *, *, #821, .T. ) ;
#7461=DIRECTION ( 'NONE',  ( -0.000000000000000000, -1.000000000000000000, -0.000000000000000000 ) ) ;
#7462=VECTOR ( 'NONE', #6925, 1000.000000000000000 ) ;
#7476=CARTESIAN_POINT ( 'NONE',  ( -37.50000000000002132, -6.000000000000000000, 24.99999999999998224 ) ) ;
#7479=FACE_OUTER_BOUND ( 'NONE', #1600, .T. ) ;
#7518=CIRCLE ( 'NONE', #15654, 2.999999999999999112 ) ;
#7545=DIRECTION ( 'NONE',  ( 0.000000000000000000, -0.000000000000000000, -1.000000000000000000 ) ) ;
#7550=AXIS2_PLACEMENT_3D ( 'NONE', #7615, #4581, #17808 ) ;
#7551=DIRECTION ( 'NONE',  ( -0.000000000000000000, -1.000000000000000000, -0.000000000000000000 ) ) ;
#7556=EDGE_LOOP ( 'NONE', ( #9903, #4563, #6387, #6448 ) ) ;
#7587=DIRECTION ( 'NONE',  ( 1.000000000000000000, 0.000000000000000000, 9.251858538542970348E-17 ) ) ;
#7594=CARTESIAN_POINT ( 'NONE',  ( 14.99999999999998579, 73.00000000000001421, 23.99999999999997158 ) ) ;
#7612=PLANE ( 'NONE',  #19360 ) ;
#7615=CARTESIAN_POINT ( 'NONE',  ( -14.99999999999999645, 73.00000000000001421, 23.99999999999997868 ) ) ;
#7619=ORIENTED_EDGE ( 'NONE', *, *, #13231, .T. ) ;
#7646=DIRECTION ( 'NONE',  ( 1.000000000000000000, 0.000000000000000000, 0.000000000000000000 ) ) ;
#7658=FACE_OUTER_BOUND ( 'NONE', #2173, .T. ) ;
#7669=CARTESIAN_POINT ( 'NONE',  ( 24.99999999999998579, 0.000000000000000000, 47.49999999999997868 ) ) ;
#7672=ORIENTED_EDGE ( 'NONE', *, *, #15260, .F. ) ;
#7684=CARTESIAN_POINT ( 'NONE',  ( 24.99999999999998579, 0.000000000000000000, 47.49999999999997868 ) ) ;
#7691=VECTOR ( 'NONE', #479, 1000.000000000000000 ) ;
#7725=VERTEX_POINT ( 'NONE', #5898 ) ;
#7732=EDGE_LOOP ( 'NONE', ( #17142, #404, #2840, #10418 ) ) ;
#7735=DIRECTION ( 'NONE',  ( -0.000000000000000000, 1.000000000000000000, -0.000000000000000000 ) ) ;
#7736=ORIENTED_EDGE ( 'NONE', *, *, #10424, .T. ) ;
#7739=( GEOMETRIC_REPRESENTATION_CONTEXT ( 3 ) GLOBAL_UNCERTAINTY_ASSIGNED_CONTEXT ( ( #11195 ) ) GLOBAL_UNIT_ASSIGNED_CONTEXT ( ( #16965, #18138, #1862 ) ) REPRESENTATION_CONTEXT ( 'NONE', 'WORKASPACE' ) );
#7744=DIRECTION ( 'NONE',  ( -1.000000000000000000, 0.000000000000000000, -1.541976423090495633E-16 ) ) ;
#7745=ORIENTED_EDGE ( 'NONE', *, *, #7145, .T. ) ;
#7768=DIRECTION ( 'NONE',  ( -1.000000000000000000, 0.000000000000000000, 0.000000000000000000 ) ) ;
#7785=LINE ( 'NONE', #8950, #16301 ) ;
#7790=LINE ( 'NONE', #12762, #2684 ) ;
#7792=VECTOR ( 'NONE', #18687, 1000.000000000000000 ) ;
#7803=LINE ( 'NONE', #7239, #10693 ) ;
#7805=CARTESIAN_POINT ( 'NONE',  ( 44.99999999999997158, -1.285879139104706187E-16, 56.59999999999999432 ) ) ;
#7811=EDGE_CURVE ( 'NONE', #10184, #8734, #13429, .T. ) ;
#7826=CARTESIAN_POINT ( 'NONE',  ( 32.50000000000000000, -6.000000000000000000, -42.49999999999999289 ) ) ;
#7828=VERTEX_POINT ( 'NONE', #4434 ) ;
#7841=CARTESIAN_POINT ( 'NONE',  ( 34.99999999999999289, 0.000000000000000000, 42.49999999999997868 ) ) ;
#7861=EDGE_CURVE ( 'NONE', #10544, #109, #15115, .T. ) ;
#7869=EDGE_CURVE ( 'NONE', #2736, #4857, #18157, .T. ) ;
#7875=ORIENTED_EDGE ( 'NONE', *, *, #36, .T. ) ;
#7894=( NAMED_UNIT ( * ) PLANE_ANGLE_UNIT ( ) SI_UNIT ( $, .RADIAN. ) );
#7908=LINE ( 'NONE', #12400, #3730 ) ;
#7925=DIRECTION ( 'NONE',  ( 1.000000000000000000, 0.000000000000000000, 9.251858538542970348E-17 ) ) ;
#7934=CARTESIAN_POINT ( 'NONE',  ( -37.50000000000002132, 107.3545527679194436, 24.99999999999998224 ) ) ;
#7957=ORIENTED_EDGE ( 'NONE', *, *, #887, .T. ) ;
#7965=CARTESIAN_POINT ( 'NONE',  ( -50.00000000000001421, 0.000000000000000000, 59.99999999999997868 ) ) ;
#7979=ORIENTED_EDGE ( 'NONE', *, *, #6184, .F. ) ;
#7990=ADVANCED_FACE ( 'NONE', ( #9487 ), #12332, .T. ) ;
#8032=PLANE ( 'NONE',  #11543 ) ;
#8039=CARTESIAN_POINT ( 'NONE',  ( 32.50000000000000000, -6.000000000000000000, -45.00000000000000000 ) ) ;
#8043=DIRECTION ( 'NONE',  ( 0.000000000000000000, 1.000000000000000000, 0.000000000000000000 ) ) ;
#8049=CARTESIAN_POINT ( 'NONE',  ( -37.50000000000002132, 107.3545527679194436, -25.00000000000002132 ) ) ;
#8051=VERTEX_POINT ( 'NONE', #12619 ) ;
#8132=ORIENTED_EDGE ( 'NONE', *, *, #19335, .T. ) ;
#8146=VERTEX_POINT ( 'NONE', #10047 ) ;
#8149=DIRECTION ( 'NONE',  ( 0.000000000000000000, 0.000000000000000000, -1.000000000000000000 ) ) ;
#8181=FILL_AREA_STYLE ('',( #18186 ) ) ;
#8186=VECTOR ( 'NONE', #1971, 1000.000000000000000 ) ;
#8187=ORIENTED_EDGE ( 'NONE', *, *, #1225, .F. ) ;
#8194=LINE ( 'NONE', #3482, #10706 ) ;
#8196=VECTOR ( 'NONE', #13480, 1000.000000000000000 ) ;
#8209=EDGE_LOOP ( 'NONE', ( #2273, #16141, #18921, #9006 ) ) ;
#8288=CYLINDRICAL_SURFACE ( 'NONE', #6176, 1.599999999999997202 ) ;
#8300=EDGE_LOOP ( 'NONE', ( #3818, #12808, #11927, #9311, #11454, #17237 ) ) ;
#8312=EDGE_LOOP ( 'NONE', ( #5259, #17352, #2147, #2333 ) ) ;
#8329=CARTESIAN_POINT ( 'NONE',  ( 44.99999999999998579, 0.000000000000000000, -56.59999999999998010 ) ) ;
#8331=DIRECTION ( 'NONE',  ( -1.000000000000000000, 0.000000000000000000, 0.000000000000000000 ) ) ;
#8333=AXIS2_PLACEMENT_3D ( 'NONE', #2415, #12529, #8399 ) ;
#8335=EDGE_CURVE ( 'NONE', #16872, #18667, #1338, .T. ) ;
#8336=VECTOR ( 'NONE', #648, 1000.000000000000000 ) ;
#8339=PLANE ( 'NONE',  #13308 ) ;
#8358=DIRECTION ( 'NONE',  ( -1.000000000000000000, 0.000000000000000000, -1.541976423090495633E-16 ) ) ;
#8364=DIRECTION ( 'NONE',  ( 0.000000000000000000, -1.000000000000000000, 0.000000000000000000 ) ) ;
#8367=ORIENTED_EDGE ( 'NONE', *, *, #15020, .F. ) ;
#8391=DIRECTION ( 'NONE',  ( 1.000000000000000000, 0.000000000000000000, 2.973811673103096679E-16 ) ) ;
#8399=DIRECTION ( 'NONE',  ( 1.000000000000000000, 0.000000000000000000, 2.973811673103096679E-16 ) ) ;
#8400=ORIENTED_EDGE ( 'NONE', *, *, #15721, .F. ) ;
#8406=ORIENTED_EDGE ( 'NONE', *, *, #510, .F. ) ;
#8424=EDGE_CURVE ( 'NONE', #9017, #12139, #18222, .T. ) ;
#8429=ORIENTED_EDGE ( 'NONE', *, *, #423, .T. ) ;
#8432=VERTEX_POINT ( 'NONE', #15451 ) ;
#8434=AXIS2_PLACEMENT_3D ( 'NONE', #10508, #17676, #1611 ) ;
#8468=CARTESIAN_POINT ( 'NONE',  ( -44.99999999999998579, 0.000000000000000000, -56.59999999999999432 ) ) ;
#8498=ORIENTED_EDGE ( 'NONE', *, *, #13564, .F. ) ;
#8501=ORIENTED_EDGE ( 'NONE', *, *, #654, .F. ) ;
#8539=CARTESIAN_POINT ( 'NONE',  ( -50.00000000000001421, 0.000000000000000000, 59.99999999999997868 ) ) ;
#8542=PLANE ( 'NONE',  #15520 ) ;
#8565=EDGE_CURVE ( 'NONE', #16200, #16449, #11568, .T. ) ;
#8582=EDGE_CURVE ( 'NONE', #2908, #17921, #7167, .T. ) ;
#8613=AXIS2_PLACEMENT_3D ( 'NONE', #8039, #7744, #572 ) ;
#8630=VECTOR ( 'NONE', #6122, 1000.000000000000000 ) ;
#8636=DIRECTION ( 'NONE',  ( -7.709882115452476934E-17, -0.000000000000000000, -1.000000000000000000 ) ) ;
#8669=LINE ( 'NONE', #18976, #6650 ) ;
#8677=CARTESIAN_POINT ( 'NONE',  ( 32.50000000000000000, -6.000000000000000000, -42.49999999999999289 ) ) ;
#8697=PLANE ( 'NONE',  #4410 ) ;
#8706=LINE ( 'NONE', #8815, #16128 ) ;
#8708=EDGE_LOOP ( 'NONE', ( #17104, #19251 ) ) ;
#8713=ORIENTED_EDGE ( 'NONE', *, *, #5580, .T. ) ;
#8722=DIRECTION ( 'NONE',  ( -1.000000000000000000, 0.000000000000000000, 0.000000000000000000 ) ) ;
#8734=VERTEX_POINT ( 'NONE', #14718 ) ;
#8756=AXIS2_PLACEMENT_3D ( 'NONE', #13533, #6093, #10584 ) ;
#8781=ADVANCED_FACE ( 'NONE', ( #3253 ), #5900, .F. ) ;
#8808=AXIS2_PLACEMENT_3D ( 'NONE', #15470, #2409, #6922 ) ;
#8815=CARTESIAN_POINT ( 'NONE',  ( -35.00000000000002132, -0.000000000000000000, -47.50000000000002132 ) ) ;
#8821=CARTESIAN_POINT ( 'NONE',  ( -37.50000000000002132, -6.000000000000000000, -25.00000000000002132 ) ) ;
#8826=DIRECTION ( 'NONE',  ( 1.000000000000000000, 0.000000000000000000, 2.081668171172167774E-16 ) ) ;
#8852=CARTESIAN_POINT ( 'NONE',  ( -50.00000000000002132, 0.000000000000000000, -60.00000000000002132 ) ) ;
#8853=DIRECTION ( 'NONE',  ( -7.304098846218135653E-17, 0.000000000000000000, 1.000000000000000000 ) ) ;
#8893=ORIENTED_EDGE ( 'NONE', *, *, #276, .F. ) ;
#8897=EDGE_CURVE ( 'NONE', #2845, #18598, #18161, .T. ) ;
#8909=EDGE_LOOP ( 'NONE', ( #12169, #10030, #15676, #13192, #1567, #3598 ) ) ;
#8946=FACE_OUTER_BOUND ( 'NONE', #11431, .T. ) ;
#8950=CARTESIAN_POINT ( 'NONE',  ( 34.99999999999999289, 0.000000000000000000, 42.49999999999997868 ) ) ;
#8951=ADVANCED_FACE ( 'NONE', ( #3828 ), #16882, .F. ) ;
#8958=LINE ( 'NONE', #14748, #12074 ) ;
#8977=CIRCLE ( 'NONE', #9295, 2.999999999999999112 ) ;
#8985=ORIENTED_EDGE ( 'NONE', *, *, #2913, .T. ) ;
#8986=ORIENTED_EDGE ( 'NONE', *, *, #7145, .F. ) ;
#9006=ORIENTED_EDGE ( 'NONE', *, *, #124, .T. ) ;
#9015=CARTESIAN_POINT ( 'NONE',  ( 37.50000000000000711, 0.000000000000000000, -45.00000000000000000 ) ) ;
#9017=VERTEX_POINT ( 'NONE', #17261 ) ;
#9035=ORIENTED_EDGE ( 'NONE', *, *, #10033, .F. ) ;
#9041=EDGE_CURVE ( 'NONE', #4229, #2520, #12361, .T. ) ;
#9072=LINE ( 'NONE', #62, #15921 ) ;
#9073=DIRECTION ( 'NONE',  ( -0.000000000000000000, -1.000000000000000000, -0.000000000000000000 ) ) ;
#9095=VERTEX_POINT ( 'NONE', #18559 ) ;
#9112=ORIENTED_EDGE ( 'NONE', *, *, #19242, .F. ) ;
#9142=FACE_BOUND ( 'NONE', #13322, .T. ) ;
#9171=LINE ( 'NONE', #18098, #8196 ) ;
#9172=DIRECTION ( 'NONE',  ( 1.000000000000000000, 0.000000000000000000, 2.973811673103096679E-16 ) ) ;
#9202=LINE ( 'NONE', #6180, #12992 ) ;
#9207=ORIENTED_EDGE ( 'NONE', *, *, #11832, .F. ) ;
#9253=ORIENTED_EDGE ( 'NONE', *, *, #11422, .F. ) ;
#9263=AXIS2_PLACEMENT_3D ( 'NONE', #14284, #17049, #9947 ) ;
#9277=VECTOR ( 'NONE', #15886, 1000.000000000000000 ) ;
#9280=EDGE_CURVE ( 'NONE', #4229, #10346, #1165, .T. ) ;
#9287=ORIENTED_EDGE ( 'NONE', *, *, #1469, .T. ) ;
#9291=DIRECTION ( 'NONE',  ( -0.000000000000000000, -1.000000000000000000, -0.000000000000000000 ) ) ;
#9295=AXIS2_PLACEMENT_3D ( 'NONE', #16566, #4617, #11744 ) ;
#9304=SURFACE_SIDE_STYLE ('',( #9585 ) ) ;
#9311=ORIENTED_EDGE ( 'NONE', *, *, #5196, .T. ) ;
#9327=CARTESIAN_POINT ( 'NONE',  ( 32.50000000000000000, 0.000000000000000000, -45.00000000000000000 ) ) ;
#9360=CIRCLE ( 'NONE', #17820, 1.599999999999997202 ) ;
#9382=LINE ( 'NONE', #10949, #13857 ) ;
#9431=PRODUCT_DEFINITION_CONTEXT ( 'detailed design', #18841, 'design' ) ;
#9433=VECTOR ( 'NONE', #18027, 1000.000000000000000 ) ;
#9445=DIRECTION ( 'NONE',  ( 0.000000000000000000, -0.000000000000000000, -1.000000000000000000 ) ) ;
#9446=CARTESIAN_POINT ( 'NONE',  ( -25.00000000000001421, 0.000000000000000000, 42.49999999999997868 ) ) ;
#9485=CARTESIAN_POINT ( 'NONE',  ( -50.00000000000001421, 3.000000000000000000, 59.99999999999997868 ) ) ;
#9487=FACE_OUTER_BOUND ( 'NONE', #14513, .T. ) ;
#9491=ORIENTED_EDGE ( 'NONE', *, *, #4490, .F. ) ;
#9508=ORIENTED_EDGE ( 'NONE', *, *, #18880, .F. ) ;
#9509=FACE_OUTER_BOUND ( 'NONE', #17218, .T. ) ;
#9540=ADVANCED_FACE ( 'NONE', ( #13999 ), #673, .T. ) ;
#9552=CARTESIAN_POINT ( 'NONE',  ( 44.99999999999998579, 0.000000000000000000, -54.99999999999998579 ) ) ;
#9585=SURFACE_STYLE_FILL_AREA ( #14004 ) ;
#9586=ORIENTED_EDGE ( 'NONE', *, *, #11422, .T. ) ;
#9611=CARTESIAN_POINT ( 'NONE',  ( -44.99999999999998579, 0.000000000000000000, -55.00000000000000000 ) ) ;
#9615=EDGE_CURVE ( 'NONE', #16872, #14967, #3521, .T. ) ;
#9624=ORIENTED_EDGE ( 'NONE', *, *, #11494, .F. ) ;
#9630=EDGE_CURVE ( 'NONE', #109, #14590, #4901, .T. ) ;
#9663=VECTOR ( 'NONE', #9073, 1000.000000000000000 ) ;
#9667=AXIS2_PLACEMENT_3D ( 'NONE', #9552, #3677, #12597 ) ;
#9672=DIRECTION ( 'NONE',  ( -0.000000000000000000, -1.000000000000000000, -0.000000000000000000 ) ) ;
#9678=ORIENTED_EDGE ( 'NONE', *, *, #9615, .F. ) ;
#9680=VECTOR ( 'NONE', #4350, 1000.000000000000000 ) ;
#9689=CARTESIAN_POINT ( 'NONE',  ( -37.50000000000002132, 0.000000000000000000, 47.49999999999997868 ) ) ;
#9765=CARTESIAN_POINT ( 'NONE',  ( 24.99999999999998579, 107.3545527679194436, 47.49999999999997868 ) ) ;
#9781=FACE_BOUND ( 'NONE', #10507, .T. ) ;
#9791=DIRECTION ( 'NONE',  ( -2.973811673103096679E-16, 0.000000000000000000, 1.000000000000000000 ) ) ;
#9799=ORIENTED_EDGE ( 'NONE', *, *, #13664, .T. ) ;
#9812=CARTESIAN_POINT ( 'NONE',  ( -45.00000000000000000, 0.000000000000000000, 54.99999999999998579 ) ) ;
#9839=VECTOR ( 'NONE', #12872, 1000.000000000000000 ) ;
#9844=CYLINDRICAL_SURFACE ( 'NONE', #19165, 1.599999999999997202 ) ;
#9851=LINE ( 'NONE', #19075, #366 ) ;
#9859=FACE_OUTER_BOUND ( 'NONE', #19201, .T. ) ;
#9879=ORIENTED_EDGE ( 'NONE', *, *, #2327, .F. ) ;
#9881=LINE ( 'NONE', #19106, #17813 ) ;
#9893=CARTESIAN_POINT ( 'NONE',  ( -14.99999999999999645, 73.00000000000001421, 23.99999999999997868 ) ) ;
#9903=ORIENTED_EDGE ( 'NONE', *, *, #848, .F. ) ;
#9947=DIRECTION ( 'NONE',  ( -1.000000000000000000, 0.000000000000000000, 0.000000000000000000 ) ) ;
#9963=ORIENTED_EDGE ( 'NONE', *, *, #11373, .T. ) ;
#9969=DIRECTION ( 'NONE',  ( 1.000000000000000000, 0.000000000000000000, 2.973811673103096679E-16 ) ) ;
#9986=ORIENTED_EDGE ( 'NONE', *, *, #13231, .F. ) ;
#9993=VERTEX_POINT ( 'NONE', #16432 ) ;
#9995=LINE ( 'NONE', #4031, #11723 ) ;
#10009=VECTOR ( 'NONE', #13746, 1000.000000000000000 ) ;
#10015=AXIS2_PLACEMENT_3D ( 'NONE', #4632, #407, #3440 ) ;
#10030=ORIENTED_EDGE ( 'NONE', *, *, #13564, .T. ) ;
#10033=EDGE_CURVE ( 'NONE', #8432, #13561, #16004, .T. ) ;
#10037=FACE_OUTER_BOUND ( 'NONE', #2543, .T. ) ;
#10047=CARTESIAN_POINT ( 'NONE',  ( -44.99999999999998579, -1.285879139104706187E-16, -53.40000000000000568 ) ) ;
#10068=VERTEX_POINT ( 'NONE', #3375 ) ;
#10081=ORIENTED_EDGE ( 'NONE', *, *, #17357, .T. ) ;
#10146=ORIENTED_EDGE ( 'NONE', *, *, #19335, .F. ) ;
#10164=FACE_OUTER_BOUND ( 'NONE', #17147, .T. ) ;
#10184=VERTEX_POINT ( 'NONE', #15903 ) ;
#10186=DIRECTION ( 'NONE',  ( 0.000000000000000000, -0.000000000000000000, -1.000000000000000000 ) ) ;
#10209=ORIENTED_EDGE ( 'NONE', *, *, #7869, .T. ) ;
#10224=ADVANCED_FACE ( 'NONE', ( #3945 ), #3665, .F. ) ;
#10233=CARTESIAN_POINT ( 'NONE',  ( -25.00000000000000711, -6.000000000000000000, -42.50000000000001421 ) ) ;
#10246=ORIENTED_EDGE ( 'NONE', *, *, #13664, .F. ) ;
#10259=DIRECTION ( 'NONE',  ( 0.000000000000000000, 1.000000000000000000, -0.000000000000000000 ) ) ;
#10299=CIRCLE ( 'NONE', #3111, 1.599999999999997202 ) ;
#10301=VECTOR ( 'NONE', #18613, 1000.000000000000000 ) ;
#10321=VECTOR ( 'NONE', #10603, 1000.000000000000000 ) ;
#10336=AXIS2_PLACEMENT_3D ( 'NONE', #12151, #3435, #5013 ) ;
#10346=VERTEX_POINT ( 'NONE', #4924 ) ;
#10351=DIRECTION ( 'NONE',  ( 1.000000000000000000, 0.000000000000000000, 2.973811673103096679E-16 ) ) ;
#10364=DIRECTION ( 'NONE',  ( 0.000000000000000000, 0.000000000000000000, -1.000000000000000000 ) ) ;
#10379=PLANE ( 'NONE',  #5237 ) ;
#10398=ADVANCED_FACE ( 'NONE', ( #9509 ), #16778, .F. ) ;
#10418=ORIENTED_EDGE ( 'NONE', *, *, #2054, .T. ) ;
#10424=EDGE_CURVE ( 'NONE', #7725, #16789, #12642, .T. ) ;
#10455=EDGE_LOOP ( 'NONE', ( #8498, #8893, #2768, #18041 ) ) ;
#10474=DIRECTION ( 'NONE',  ( 1.000000000000000000, 0.000000000000000000, 9.251858538542970348E-17 ) ) ;
#10479=CARTESIAN_POINT ( 'NONE',  ( 32.49999999999998579, 0.000000000000000000, 24.99999999999998224 ) ) ;
#10486=ORIENTED_EDGE ( 'NONE', *, *, #18880, .T. ) ;
#10496=CARTESIAN_POINT ( 'NONE',  ( -25.00000000000001421, 0.000000000000000000, 47.49999999999997868 ) ) ;
#10507=EDGE_LOOP ( 'NONE', ( #9207, #3856, #14465, #17541, #17042, #10644 ) ) ;
#10508=CARTESIAN_POINT ( 'NONE',  ( 34.99999999999999289, -6.000000000000000000, 47.49999999999997868 ) ) ;
#10532=CARTESIAN_POINT ( 'NONE',  ( -32.50000000000001421, -6.000000000000000000, 44.99999999999997868 ) ) ;
#10544=VERTEX_POINT ( 'NONE', #6766 ) ;
#10561=CARTESIAN_POINT ( 'NONE',  ( -25.00000000000001421, -6.000000000000000000, 47.49999999999997868 ) ) ;
#10562=CARTESIAN_POINT ( 'NONE',  ( 24.99999999999999289, 107.3545527679194436, -47.50000000000002132 ) ) ;
#10571=CARTESIAN_POINT ( 'NONE',  ( -25.00000000000000711, 0.000000000000000000, -47.50000000000002132 ) ) ;
#10576=EDGE_CURVE ( 'NONE', #14588, #2736, #7803, .T. ) ;
#10579=ORIENTED_EDGE ( 'NONE', *, *, #18638, .F. ) ;
#10584=DIRECTION ( 'NONE',  ( -1.156482317317871725E-16, 0.000000000000000000, 1.000000000000000000 ) ) ;
#10603=DIRECTION ( 'NONE',  ( 1.000000000000000000, 0.000000000000000000, 2.973811673103096679E-16 ) ) ;
#10608=PLANE ( 'NONE',  #18326 ) ;
#10615=VECTOR ( 'NONE', #1066, 1000.000000000000000 ) ;
#10642=AXIS2_PLACEMENT_3D ( 'NONE', #9611, #2077, #12739 ) ;
#10644=ORIENTED_EDGE ( 'NONE', *, *, #8582, .F. ) ;
#10665=ORIENTED_EDGE ( 'NONE', *, *, #19337, .T. ) ;
#10669=SURFACE_STYLE_USAGE ( .BOTH. , #9304 ) ;
#10675=EDGE_CURVE ( 'NONE', #6389, #13623, #252, .T. ) ;
#10682=AXIS2_PLACEMENT_3D ( 'NONE', #4671, #4377, #13182 ) ;
#10689=CARTESIAN_POINT ( 'NONE',  ( -32.50000000000001421, -6.000000000000000000, 44.99999999999997868 ) ) ;
#10692=CARTESIAN_POINT ( 'NONE',  ( -45.00000000000000000, 0.000000000000000000, 53.39999999999999147 ) ) ;
#10693=VECTOR ( 'NONE', #19202, 1000.000000000000000 ) ;
#10700=DIRECTION ( 'NONE',  ( 0.000000000000000000, 0.000000000000000000, -1.000000000000000000 ) ) ;
#10701=ORIENTED_EDGE ( 'NONE', *, *, #19242, .T. ) ;
#10704=CARTESIAN_POINT ( 'NONE',  ( 0.000000000000000000, 0.000000000000000000, 0.000000000000000000 ) ) ;
#10706=VECTOR ( 'NONE', #18491, 1000.000000000000000 ) ;
#10709=CARTESIAN_POINT ( 'NONE',  ( 14.99999999999998579, 73.00000000000001421, 20.99999999999997513 ) ) ;
#10712=DIRECTION ( 'NONE',  ( -1.541976423090495880E-16, 0.000000000000000000, 1.000000000000000000 ) ) ;
#10713=DIRECTION ( 'NONE',  ( -0.000000000000000000, -1.000000000000000000, -0.000000000000000000 ) ) ;
#10714=FACE_BOUND ( 'NONE', #17420, .T. ) ;
#10719=DIRECTION ( 'NONE',  ( 0.000000000000000000, 0.000000000000000000, -1.000000000000000000 ) ) ;
#10730=DIRECTION ( 'NONE',  ( -0.000000000000000000, -1.000000000000000000, -0.000000000000000000 ) ) ;
#10748=LINE ( 'NONE', #17926, #5400 ) ;
#10761=VERTEX_POINT ( 'NONE', #4205 ) ;
#10764=ORIENTED_EDGE ( 'NONE', *, *, #7308, .T. ) ;
#10767=( GEOMETRIC_REPRESENTATION_CONTEXT ( 3 ) GLOBAL_UNCERTAINTY_ASSIGNED_CONTEXT ( ( #2192 ) ) GLOBAL_UNIT_ASSIGNED_CONTEXT ( ( #3374, #7894, #15529 ) ) REPRESENTATION_CONTEXT ( 'NONE', 'WORKASPACE' ) );
#10782=PLANE ( 'NONE',  #17115 ) ;
#10788=VECTOR ( 'NONE', #10712, 1000.000000000000000 ) ;
#10812=VECTOR ( 'NONE', #6206, 1000.000000000000000 ) ;
#10831=EDGE_CURVE ( 'NONE', #7725, #17240, #8669, .T. ) ;
#10834=DIRECTION ( 'NONE',  ( 0.000000000000000000, 1.000000000000000000, -0.000000000000000000 ) ) ;
#10858=LINE ( 'NONE', #9485, #15641 ) ;
#10859=CIRCLE ( 'NONE', #15570, 1.599999999999997202 ) ;
#10861=DIRECTION ( 'NONE',  ( -0.000000000000000000, 1.000000000000000000, -0.000000000000000000 ) ) ;
#10863=VERTEX_POINT ( 'NONE', #5546 ) ;
#10864=ORIENTED_EDGE ( 'NONE', *, *, #17785, .T. ) ;
#10865=EDGE_LOOP ( 'NONE', ( #2317, #320, #10246, #6092 ) ) ;
#10879=EDGE_LOOP ( 'NONE', ( #11664, #15285, #5014, #1557 ) ) ;
#10883=CARTESIAN_POINT ( 'NONE',  ( -32.50000000000002132, -6.000000000000000000, -25.00000000000002842 ) ) ;
#10894=ADVANCED_FACE ( 'NONE', ( #10037 ), #9844, .F. ) ;
#10900=VERTEX_POINT ( 'NONE', #10233 ) ;
#10911=CYLINDRICAL_SURFACE ( 'NONE', #1130, 2.999999999999999112 ) ;
#10920=CARTESIAN_POINT ( 'NONE',  ( -45.00000000000000000, 3.000000000000000000, 54.99999999999998579 ) ) ;
#10936=VECTOR ( 'NONE', #14635, 1000.000000000000000 ) ;
#10949=CARTESIAN_POINT ( 'NONE',  ( -25.00000000000000711, 107.3545527679194436, -47.50000000000002132 ) ) ;
#10957=LINE ( 'NONE', #6270, #7691 ) ;
#10977=CARTESIAN_POINT ( 'NONE',  ( -37.50000000000002842, -6.000000000000000000, -47.50000000000002132 ) ) ;
#11006=FACE_BOUND ( 'NONE', #12641, .T. ) ;
#11031=EDGE_LOOP ( 'NONE', ( #17941, #16505, #10764, #6990 ) ) ;
#11046=CARTESIAN_POINT ( 'NONE',  ( 32.49999999999998579, -6.000000000000000000, 42.49999999999997868 ) ) ;
#11054=ADVANCED_FACE ( 'NONE', ( #9781, #686, #6755, #6670, #15774, #12633, #18812, #9142, #18630 ), #5386, .T. ) ;
#11140=DIRECTION ( 'NONE',  ( 1.000000000000000000, 0.000000000000000000, 0.000000000000000000 ) ) ;
#11149=ORIENTED_EDGE ( 'NONE', *, *, #5697, .T. ) ;
#11157=EDGE_LOOP ( 'NONE', ( #1501, #8132, #7238, #14570 ) ) ;
#11160=CARTESIAN_POINT ( 'NONE',  ( -50.00000000000002132, 3.000000000000000000, -60.00000000000002132 ) ) ;
#11161=ORIENTED_EDGE ( 'NONE', *, *, #4354, .F. ) ;
#11190=EDGE_CURVE ( 'NONE', #2533, #10900, #5472, .T. ) ;
#11195=UNCERTAINTY_MEASURE_WITH_UNIT (LENGTH_MEASURE( 1.000000000000000082E-05 ), #16965, 'distance_accuracy_value', 'NONE');
#11200=DIRECTION ( 'NONE',  ( -0.000000000000000000, -1.000000000000000000, -0.000000000000000000 ) ) ;
#11224=PLANE ( 'NONE',  #1302 ) ;
#11230=AXIS2_PLACEMENT_3D ( 'NONE', #17849, #4422, #4623 ) ;
#11231=CARTESIAN_POINT ( 'NONE',  ( -37.50000000000002132, 0.000000000000000000, 24.99999999999998224 ) ) ;
#11281=PLANE ( 'NONE',  #7364 ) ;
#11295=VECTOR ( 'NONE', #6202, 1000.000000000000000 ) ;
#11323=EDGE_CURVE ( 'NONE', #5562, #15859, #16353, .T. ) ;
#11325=VECTOR ( 'NONE', #5934, 1000.000000000000000 ) ;
#11331=VECTOR ( 'NONE', #7735, 1000.000000000000000 ) ;
#11339=ORIENTED_EDGE ( 'NONE', *, *, #17357, .F. ) ;
#11343=DIRECTION ( 'NONE',  ( 0.000000000000000000, -0.000000000000000000, -1.000000000000000000 ) ) ;
#11359=ORIENTED_EDGE ( 'NONE', *, *, #14999, .F. ) ;
#11373=EDGE_CURVE ( 'NONE', #13561, #19091, #10748, .T. ) ;
#11380=CARTESIAN_POINT ( 'NONE',  ( 32.50000000000000000, 0.000000000000000000, -42.49999999999999289 ) ) ;
#11422=EDGE_CURVE ( 'NONE', #18257, #10863, #12197, .T. ) ;
#11431=EDGE_LOOP ( 'NONE', ( #1858, #7672, #3213, #11339 ) ) ;
#11454=ORIENTED_EDGE ( 'NONE', *, *, #4372, .T. ) ;
#11471=COLOUR_RGB ( '', 0.40784314, 0.44705882, 0.49803922) ;
#11494=EDGE_CURVE ( 'NONE', #3455, #13355, #15342, .T. ) ;
#11499=EDGE_CURVE ( 'NONE', #17265, #11522, #8194, .T. ) ;
#11514=EDGE_CURVE ( 'NONE', #2416, #717, #13200, .T. ) ;
#11516=ORIENTED_EDGE ( 'NONE', *, *, #14751, .F. ) ;
#11522=VERTEX_POINT ( 'NONE', #3383 ) ;
#11537=VECTOR ( 'NONE', #7211, 1000.000000000000000 ) ;
#11543=AXIS2_PLACEMENT_3D ( 'NONE', #5270, #2233, #6461 ) ;
#11550=CARTESIAN_POINT ( 'NONE',  ( 37.49999999999999289, -6.000000000000000000, -25.00000000000001421 ) ) ;
#11561=ORIENTED_EDGE ( 'NONE', *, *, #18557, .T. ) ;
#11568=LINE ( 'NONE', #16003, #17277 ) ;
#11651=DIRECTION ( 'NONE',  ( -0.000000000000000000, -1.000000000000000000, -0.000000000000000000 ) ) ;
#11664=ORIENTED_EDGE ( 'NONE', *, *, #4011, .T. ) ;
#11665=CARTESIAN_POINT ( 'NONE',  ( -44.99999999999998579, 0.000000000000000000, -53.40000000000000568 ) ) ;
#11667=DIRECTION ( 'NONE',  ( 0.000000000000000000, -0.000000000000000000, -1.000000000000000000 ) ) ;
#11723=VECTOR ( 'NONE', #16000, 1000.000000000000000 ) ;
#11729=ORIENTED_EDGE ( 'NONE', *, *, #18972, .T. ) ;
#11739=DIRECTION ( 'NONE',  ( -1.000000000000000000, 0.000000000000000000, -0.000000000000000000 ) ) ;
#11742=VERTEX_POINT ( 'NONE', #6991 ) ;
#11744=DIRECTION ( 'NONE',  ( 0.000000000000000000, 0.000000000000000000, 1.000000000000000000 ) ) ;
#11745=ORIENTED_EDGE ( 'NONE', *, *, #124, .F. ) ;
#11746=ORIENTED_EDGE ( 'NONE', *, *, #11190, .F. ) ;
#11753=AXIS2_PLACEMENT_3D ( 'NONE', #3567, #14053, #3206 ) ;
#11762=CARTESIAN_POINT ( 'NONE',  ( 49.99999999999998579, 0.000000000000000000, 59.99999999999997868 ) ) ;
#11827=ORIENTED_EDGE ( 'NONE', *, *, #17785, .F. ) ;
#11830=LINE ( 'NONE', #1359, #11331 ) ;
#11832=EDGE_CURVE ( 'NONE', #18667, #2908, #6215, .T. ) ;
#11840=ORIENTED_EDGE ( 'NONE', *, *, #5697, .F. ) ;
#11844=VERTEX_POINT ( 'NONE', #7476 ) ;
#11869=VECTOR ( 'NONE', #14704, 1000.000000000000000 ) ;
#11871=EDGE_LOOP ( 'NONE', ( #11746, #6835, #17974, #3836 ) ) ;
#11911=DIRECTION ( 'NONE',  ( -0.000000000000000000, -1.000000000000000000, -0.000000000000000000 ) ) ;
#11927=ORIENTED_EDGE ( 'NONE', *, *, #13679, .T. ) ;
#11939=CARTESIAN_POINT ( 'NONE',  ( -25.00000000000001421, 107.3545527679194436, 47.49999999999997868 ) ) ;
#11940=DIRECTION ( 'NONE',  ( -0.000000000000000000, 1.000000000000000000, -0.000000000000000000 ) ) ;
#11942=LINE ( 'NONE', #3021, #14361 ) ;
#11964=DIRECTION ( 'NONE',  ( -0.000000000000000000, -1.000000000000000000, -0.000000000000000000 ) ) ;
#11969=CIRCLE ( 'NONE', #18248, 2.999999999999999112 ) ;
#11986=CARTESIAN_POINT ( 'NONE',  ( -45.00000000000000000, -1.285879139104706187E-16, 54.99999999999998579 ) ) ;
#12006=CARTESIAN_POINT ( 'NONE',  ( -25.00000000000001421, 0.000000000000000000, 47.49999999999997868 ) ) ;
#12030=CARTESIAN_POINT ( 'NONE',  ( 24.99999999999998579, -6.000000000000000000, 47.49999999999997868 ) ) ;
#12040=DIRECTION ( 'NONE',  ( -0.000000000000000000, -1.000000000000000000, -0.000000000000000000 ) ) ;
#12046=CARTESIAN_POINT ( 'NONE',  ( -44.99999999999998579, 3.000000000000000000, -53.40000000000000568 ) ) ;
#12049=EDGE_LOOP ( 'NONE', ( #2454, #13796, #3269, #4089 ) ) ;
#12074=VECTOR ( 'NONE', #14947, 1000.000000000000000 ) ;
#12082=CARTESIAN_POINT ( 'NONE',  ( -14.99999999999999645, 73.00000000000001421, 20.99999999999998224 ) ) ;
#12096=STYLED_ITEM ( 'NONE', ( #12438 ), #571 ) ;
#12139=VERTEX_POINT ( 'NONE', #10709 ) ;
#12143=FILL_AREA_STYLE_COLOUR ( '', #11471 ) ;
#12151=CARTESIAN_POINT ( 'NONE',  ( -50.00000000000001421, 3.000000000000000000, 59.99999999999997868 ) ) ;
#12157=CARTESIAN_POINT ( 'NONE',  ( -14.99999999999999645, 3.000000000000000000, 26.99999999999997868 ) ) ;
#12166=ORIENTED_EDGE ( 'NONE', *, *, #1242, .F. ) ;
#12169=ORIENTED_EDGE ( 'NONE', *, *, #19065, .T. ) ;
#12180=EDGE_LOOP ( 'NONE', ( #10146, #2611, #13915, #9287, #5389, #18657 ) ) ;
#12184=PLANE ( 'NONE',  #273 ) ;
#12188=CARTESIAN_POINT ( 'NONE',  ( 32.50000000000000000, -6.000000000000000000, -25.00000000000001421 ) ) ;
#12197=LINE ( 'NONE', #19365, #11325 ) ;
#12212=ORIENTED_EDGE ( 'NONE', *, *, #12280, .T. ) ;
#12227=EDGE_CURVE ( 'NONE', #18340, #10184, #18847, .T. ) ;
#12228=CARTESIAN_POINT ( 'NONE',  ( -35.00000000000002132, -6.000000000000000000, -42.50000000000001421 ) ) ;
#12240=PLANE ( 'NONE',  #8613 ) ;
#12241=EDGE_LOOP ( 'NONE', ( #7619, #13330 ) ) ;
#12245=VECTOR ( 'NONE', #15215, 1000.000000000000000 ) ;
#12257=VECTOR ( 'NONE', #5455, 1000.000000000000000 ) ;
#12267=VECTOR ( 'NONE', #8636, 1000.000000000000000 ) ;
#12280=EDGE_CURVE ( 'NONE', #13683, #5958, #10299, .T. ) ;
#12295=LINE ( 'NONE', #12188, #8630 ) ;
#12313=CARTESIAN_POINT ( 'NONE',  ( -32.50000000000001421, 0.000000000000000000, 42.49999999999997868 ) ) ;
#12332=PLANE ( 'NONE',  #16952 ) ;
#12333=DIRECTION ( 'NONE',  ( 1.000000000000000000, 0.000000000000000000, -7.709882115452476934E-17 ) ) ;
#12353=DIRECTION ( 'NONE',  ( -7.304098846218135653E-17, 0.000000000000000000, 1.000000000000000000 ) ) ;
#12360=FACE_OUTER_BOUND ( 'NONE', #394, .T. ) ;
#12361=LINE ( 'NONE', #18735, #3773 ) ;
#12364=AXIS2_PLACEMENT_3D ( 'NONE', #10920, #13871, #14164 ) ;
#12367=EDGE_CURVE ( 'NONE', #109, #6502, #4137, .T. ) ;
#12376=ORIENTED_EDGE ( 'NONE', *, *, #13319, .T. ) ;
#12379=ORIENTED_EDGE ( 'NONE', *, *, #5680, .T. ) ;
#12382=DIRECTION ( 'NONE',  ( -1.541976423090495880E-16, 0.000000000000000000, 1.000000000000000000 ) ) ;
#12387=SURFACE_SIDE_STYLE ('',( #14049 ) ) ;
#12400=CARTESIAN_POINT ( 'NONE',  ( 32.50000000000000000, 0.000000000000000000, -45.00000000000000000 ) ) ;
#12402=ADVANCED_FACE ( 'NONE', ( #19130 ), #16181, .F. ) ;
#12430=AXIS2_PLACEMENT_3D ( 'NONE', #9893, #795, #5307 ) ;
#12438=PRESENTATION_STYLE_ASSIGNMENT (( #10669 ) ) ;
#12451=CARTESIAN_POINT ( 'NONE',  ( 44.99999999999998579, 3.000000000000000000, -54.99999999999998579 ) ) ;
#12496=ADVANCED_FACE ( 'NONE', ( #2946 ), #14915, .F. ) ;
#12505=ORIENTED_EDGE ( 'NONE', *, *, #18977, .T. ) ;
#12511=ORIENTED_EDGE ( 'NONE', *, *, #15879, .T. ) ;
#12520=ADVANCED_FACE ( 'NONE', ( #10 ), #15008, .F. ) ;
#12528=CARTESIAN_POINT ( 'NONE',  ( -32.50000000000001421, -6.000000000000000000, 44.99999999999997868 ) ) ;
#12529=DIRECTION ( 'NONE',  ( -2.973811673103096679E-16, 0.000000000000000000, 1.000000000000000000 ) ) ;
#12530=EDGE_CURVE ( 'NONE', #12139, #9017, #7518, .T. ) ;
#12554=DIRECTION ( 'NONE',  ( 0.000000000000000000, 1.000000000000000000, 0.000000000000000000 ) ) ;
#12567=VECTOR ( 'NONE', #10861, 1000.000000000000000 ) ;
#12581=LINE ( 'NONE', #3753, #3477 ) ;
#12594=ADVANCED_FACE ( 'NONE', ( #7658 ), #16776, .F. ) ;
#12597=DIRECTION ( 'NONE',  ( 0.000000000000000000, 0.000000000000000000, -1.000000000000000000 ) ) ;
#12619=CARTESIAN_POINT ( 'NONE',  ( 24.99999999999999289, 0.000000000000000000, -47.50000000000002132 ) ) ;
#12624=DIRECTION ( 'NONE',  ( -1.000000000000000000, 0.000000000000000000, -9.251858538542970348E-17 ) ) ;
#12630=VERTEX_POINT ( 'NONE', #13624 ) ;
#12633=FACE_BOUND ( 'NONE', #8708, .T. ) ;
#12641=EDGE_LOOP ( 'NONE', ( #11729, #12511 ) ) ;
#12642=LINE ( 'NONE', #18447, #18835 ) ;
#12646=CARTESIAN_POINT ( 'NONE',  ( 44.99999999999997158, 3.000000000000000000, 55.00000000000000000 ) ) ;
#12657=MECHANICAL_DESIGN_GEOMETRIC_PRESENTATION_REPRESENTATION('',(#6416),#10767);
#12718=ORIENTED_EDGE ( 'NONE', *, *, #19065, .F. ) ;
#12739=DIRECTION ( 'NONE',  ( 0.000000000000000000, 0.000000000000000000, -1.000000000000000000 ) ) ;
#12762=CARTESIAN_POINT ( 'NONE',  ( -37.50000000000002132, -6.000000000000000000, 24.99999999999998224 ) ) ;
#12783=EDGE_LOOP ( 'NONE', ( #11516, #15110, #6661, #15221, #9491, #4649 ) ) ;
#12794=DIRECTION ( 'NONE',  ( -1.000000000000000000, 0.000000000000000000, -7.304098846218135653E-17 ) ) ;
#12808=ORIENTED_EDGE ( 'NONE', *, *, #15721, .T. ) ;
#12823=DIRECTION ( 'NONE',  ( 9.251858538542970348E-17, 0.000000000000000000, -1.000000000000000000 ) ) ;
#12833=ORIENTED_EDGE ( 'NONE', *, *, #526, .T. ) ;
#12834=EDGE_LOOP ( 'NONE', ( #9624, #9986, #13725, #12833 ) ) ;
#12846=PRODUCT ( 'Removable Bottom Crumb Tray', 'Removable Bottom Crumb Tray', '', ( #3052 ) ) ;
#12851=AXIS2_PLACEMENT_3D ( 'NONE', #11986, #10713, #4555 ) ;
#12853=EDGE_CURVE ( 'NONE', #5207, #5173, #5574, .T. ) ;
#12872=DIRECTION ( 'NONE',  ( -0.000000000000000000, -1.000000000000000000, -0.000000000000000000 ) ) ;
#12900=CARTESIAN_POINT ( 'NONE',  ( -37.50000000000002132, 0.000000000000000000, 24.99999999999998224 ) ) ;
#12905=ORIENTED_EDGE ( 'NONE', *, *, #13689, .F. ) ;
#12917=DIRECTION ( 'NONE',  ( -0.000000000000000000, -1.000000000000000000, -0.000000000000000000 ) ) ;
#12928=EDGE_LOOP ( 'NONE', ( #5318, #12379, #4817, #5016 ) ) ;
#12941=FACE_OUTER_BOUND ( 'NONE', #14928, .T. ) ;
#12992=VECTOR ( 'NONE', #12040, 1000.000000000000000 ) ;
#13013=CIRCLE ( 'NONE', #14926, 1.599999999999997202 ) ;
#13016=DIRECTION ( 'NONE',  ( 5.782411586589357392E-17, -0.000000000000000000, 1.000000000000000000 ) ) ;
#13035=DIRECTION ( 'NONE',  ( -1.000000000000000000, 0.000000000000000000, 0.000000000000000000 ) ) ;
#13107=CARTESIAN_POINT ( 'NONE',  ( 24.99999999999998579, -6.000000000000000000, 47.49999999999997868 ) ) ;
#13112=VECTOR ( 'NONE', #15713, 1000.000000000000000 ) ;
#13131=CARTESIAN_POINT ( 'NONE',  ( 14.99999999999998579, 73.00000000000001421, 23.99999999999997158 ) ) ;
#13146=ORIENTED_EDGE ( 'NONE', *, *, #526, .F. ) ;
#13171=ORIENTED_EDGE ( 'NONE', *, *, #1921, .F. ) ;
#13182=DIRECTION ( 'NONE',  ( 0.000000000000000000, 0.000000000000000000, -1.000000000000000000 ) ) ;
#13192=ORIENTED_EDGE ( 'NONE', *, *, #10576, .F. ) ;
#13200=CIRCLE ( 'NONE', #7270, 1.599999999999997202 ) ;
#13201=DIRECTION ( 'NONE',  ( 0.000000000000000000, -1.000000000000000000, 0.000000000000000000 ) ) ;
#13231=EDGE_CURVE ( 'NONE', #2845, #3455, #4219, .T. ) ;
#13232=DIRECTION ( 'NONE',  ( 9.251858538542970348E-17, 0.000000000000000000, -1.000000000000000000 ) ) ;
#13252=VERTEX_POINT ( 'NONE', #2298 ) ;
#13254=DIRECTION ( 'NONE',  ( -1.000000000000000000, 0.000000000000000000, -7.304098846218135653E-17 ) ) ;
#13263=ORIENTED_EDGE ( 'NONE', *, *, #4011, .F. ) ;
#13267=DIRECTION ( 'NONE',  ( 0.000000000000000000, 0.000000000000000000, -1.000000000000000000 ) ) ;
#13272=CARTESIAN_POINT ( 'NONE',  ( -44.99999999999998579, -1.285879139104706187E-16, -56.59999999999999432 ) ) ;
#13277=VECTOR ( 'NONE', #7587, 1000.000000000000000 ) ;
#13289=CARTESIAN_POINT ( 'NONE',  ( 32.50000000000000000, -6.000000000000000000, -45.00000000000000000 ) ) ;
#13308=AXIS2_PLACEMENT_3D ( 'NONE', #17734, #16639, #18106 ) ;
#13309=FACE_OUTER_BOUND ( 'NONE', #8209, .T. ) ;
#13319=EDGE_CURVE ( 'NONE', #9095, #628, #4052, .T. ) ;
#13322=EDGE_LOOP ( 'NONE', ( #9112, #4518 ) ) ;
#13330=ORIENTED_EDGE ( 'NONE', *, *, #19117, .T. ) ;
#13343=EDGE_LOOP ( 'NONE', ( #2942, #7957, #19298, #8429 ) ) ;
#13355=VERTEX_POINT ( 'NONE', #7090 ) ;
#13395=EDGE_LOOP ( 'NONE', ( #4136, #11149, #18169, #12905 ) ) ;
#13412=LINE ( 'NONE', #8821, #6173 ) ;
#13419=ORIENTED_EDGE ( 'NONE', *, *, #16305, .F. ) ;
#13425=DIRECTION ( 'NONE',  ( -1.000000000000000000, 0.000000000000000000, -9.251858538542970348E-17 ) ) ;
#13429=LINE ( 'NONE', #11762, #5984 ) ;
#13432=DIRECTION ( 'NONE',  ( 0.000000000000000000, 0.000000000000000000, -1.000000000000000000 ) ) ;
#13480=DIRECTION ( 'NONE',  ( -1.541976423090495880E-16, 0.000000000000000000, 1.000000000000000000 ) ) ;
#13533=CARTESIAN_POINT ( 'NONE',  ( 49.99999999999998579, 3.000000000000000000, 59.99999999999997868 ) ) ;
#13560=DIRECTION ( 'NONE',  ( -0.000000000000000000, -1.000000000000000000, -0.000000000000000000 ) ) ;
#13561=VERTEX_POINT ( 'NONE', #12082 ) ;
#13564=EDGE_CURVE ( 'NONE', #11844, #4857, #3274, .T. ) ;
#13576=CARTESIAN_POINT ( 'NONE',  ( -32.50000000000001421, -6.000000000000000000, 44.99999999999997868 ) ) ;
#13604=PLANE ( 'NONE',  #4044 ) ;
#13610=ORIENTED_EDGE ( 'NONE', *, *, #15020, .T. ) ;
#13623=VERTEX_POINT ( 'NONE', #2875 ) ;
#13624=CARTESIAN_POINT ( 'NONE',  ( 44.99999999999998579, -1.285879139104706187E-16, -53.39999999999999147 ) ) ;
#13638=CARTESIAN_POINT ( 'NONE',  ( -37.50000000000002132, 0.000000000000000000, 24.99999999999998224 ) ) ;
#13648=ORIENTED_EDGE ( 'NONE', *, *, #10576, .T. ) ;
#13651=DIRECTION ( 'NONE',  ( -1.000000000000000000, 0.000000000000000000, 0.000000000000000000 ) ) ;
#13659=ADVANCED_FACE ( 'NONE', ( #7479 ), #10608, .T. ) ;
#13664=EDGE_CURVE ( 'NONE', #10761, #17265, #4552, .T. ) ;
#13679=EDGE_CURVE ( 'NONE', #1168, #18345, #4458, .T. ) ;
#13683=VERTEX_POINT ( 'NONE', #5917 ) ;
#13689=EDGE_CURVE ( 'NONE', #12139, #428, #14838, .T. ) ;
#13694=ORIENTED_EDGE ( 'NONE', *, *, #12853, .T. ) ;
#13707=DIRECTION ( 'NONE',  ( -0.000000000000000000, -1.000000000000000000, -0.000000000000000000 ) ) ;
#13713=CARTESIAN_POINT ( 'NONE',  ( 0.000000000000000000, 0.000000000000000000, 0.000000000000000000 ) ) ;
#13725=ORIENTED_EDGE ( 'NONE', *, *, #8897, .T. ) ;
#13746=DIRECTION ( 'NONE',  ( -1.000000000000000000, 0.000000000000000000, 0.000000000000000000 ) ) ;
#13754=FACE_BOUND ( 'NONE', #561, .T. ) ;
#13796=ORIENTED_EDGE ( 'NONE', *, *, #8565, .T. ) ;
#13828=DIRECTION ( 'NONE',  ( 1.000000000000000000, 0.000000000000000000, -7.709882115452476934E-17 ) ) ;
#13851=ORIENTED_EDGE ( 'NONE', *, *, #9280, .F. ) ;
#13857=VECTOR ( 'NONE', #15376, 1000.000000000000000 ) ;
#13868=CARTESIAN_POINT ( 'NONE',  ( 44.99999999999997158, -1.285879139104706187E-16, 55.00000000000000000 ) ) ;
#13871=DIRECTION ( 'NONE',  ( 0.000000000000000000, -1.000000000000000000, 0.000000000000000000 ) ) ;
#13886=ORIENTED_EDGE ( 'NONE', *, *, #10675, .F. ) ;
#13906=SHAPE_REPRESENTATION ( 'Removable Bottom Crumb Tray', ( #1791 ), #5851 ) ;
#13914=DIRECTION ( 'NONE',  ( 1.000000000000000000, 0.000000000000000000, 2.973811673103096679E-16 ) ) ;
#13915=ORIENTED_EDGE ( 'NONE', *, *, #384, .F. ) ;
#13934=VECTOR ( 'NONE', #17883, 1000.000000000000000 ) ;
#13940=ORIENTED_EDGE ( 'NONE', *, *, #6802, .T. ) ;
#13945=EDGE_LOOP ( 'NONE', ( #9035, #577, #2491, #18997 ) ) ;
#13955=ADVANCED_FACE ( 'NONE', ( #12941 ), #11281, .T. ) ;
#13988=CARTESIAN_POINT ( 'NONE',  ( 32.49999999999998579, 0.000000000000000000, 42.49999999999997868 ) ) ;
#13994=LINE ( 'NONE', #12228, #15665 ) ;
#13999=FACE_OUTER_BOUND ( 'NONE', #15893, .T. ) ;
#14004=FILL_AREA_STYLE ('',( #12143 ) ) ;
#14010=DIRECTION ( 'NONE',  ( 0.000000000000000000, -1.000000000000000000, 0.000000000000000000 ) ) ;
#14024=ADVANCED_FACE ( 'NONE', ( #18753 ), #1183, .F. ) ;
#14027=EDGE_CURVE ( 'NONE', #16466, #10068, #9995, .T. ) ;
#14033=ADVANCED_FACE ( 'NONE', ( #18850 ), #1087, .F. ) ;
#14034=LINE ( 'NONE', #9327, #16493 ) ;
#14037=ADVANCED_FACE ( 'NONE', ( #2561 ), #8542, .T. ) ;
#14042=ORIENTED_EDGE ( 'NONE', *, *, #1596, .F. ) ;
#14049=SURFACE_STYLE_FILL_AREA ( #8181 ) ;
#14053=DIRECTION ( 'NONE',  ( -2.973811673103096679E-16, 0.000000000000000000, 1.000000000000000000 ) ) ;
#14061=DIRECTION ( 'NONE',  ( -0.000000000000000000, -1.000000000000000000, -0.000000000000000000 ) ) ;
#14106=VERTEX_POINT ( 'NONE', #12157 ) ;
#14107=ORIENTED_EDGE ( 'NONE', *, *, #5891, .F. ) ;
#14128=DIRECTION ( 'NONE',  ( -0.000000000000000000, -1.000000000000000000, -0.000000000000000000 ) ) ;
#14145=CARTESIAN_POINT ( 'NONE',  ( 24.99999999999998579, -6.000000000000000000, 42.49999999999997868 ) ) ;
#14151=DIRECTION ( 'NONE',  ( 0.000000000000000000, 0.000000000000000000, -1.000000000000000000 ) ) ;
#14154=UNCERTAINTY_MEASURE_WITH_UNIT (LENGTH_MEASURE( 1.000000000000000082E-05 ), #15196, 'distance_accuracy_value', 'NONE');
#14164=DIRECTION ( 'NONE',  ( 0.000000000000000000, 0.000000000000000000, -1.000000000000000000 ) ) ;
#14170=CARTESIAN_POINT ( 'NONE',  ( -37.50000000000002132, 0.000000000000000000, 44.99999999999997868 ) ) ;
#14193=EDGE_CURVE ( 'NONE', #10900, #1798, #16486, .T. ) ;
#14226=CYLINDRICAL_SURFACE ( 'NONE', #12430, 2.999999999999999112 ) ;
#14227=ORIENTED_EDGE ( 'NONE', *, *, #1596, .T. ) ;
#14277=LINE ( 'NONE', #3982, #12257 ) ;
#14284=CARTESIAN_POINT ( 'NONE',  ( 34.99999999999999289, -6.000000000000000000, 42.49999999999997868 ) ) ;
#14326=CARTESIAN_POINT ( 'NONE',  ( 44.99999999999997158, 3.000000000000000000, 55.00000000000000000 ) ) ;
#14361=VECTOR ( 'NONE', #16252, 1000.000000000000000 ) ;
#14372=LINE ( 'NONE', #11231, #16143 ) ;
#14407=CARTESIAN_POINT ( 'NONE',  ( -14.99999999999999645, 3.000000000000000000, 20.99999999999998224 ) ) ;
#14424=DIRECTION ( 'NONE',  ( -0.000000000000000000, 0.000000000000000000, -1.000000000000000000 ) ) ;
#14430=CARTESIAN_POINT ( 'NONE',  ( -45.00000000000000000, 0.000000000000000000, 54.99999999999998579 ) ) ;
#14456=VECTOR ( 'NONE', #13201, 1000.000000000000000 ) ;
#14465=ORIENTED_EDGE ( 'NONE', *, *, #9615, .T. ) ;
#14513=EDGE_LOOP ( 'NONE', ( #10579, #6742, #8400, #14614 ) ) ;
#14514=DIRECTION ( 'NONE',  ( 0.000000000000000000, -1.000000000000000000, 0.000000000000000000 ) ) ;
#14516=CYLINDRICAL_SURFACE ( 'NONE', #945, 2.999999999999999112 ) ;
#14517=CARTESIAN_POINT ( 'NONE',  ( 0.000000000000000000, -6.000000000000000000, 0.000000000000000000 ) ) ;
#14527=ADVANCED_FACE ( 'NONE', ( #7324 ), #16541, .T. ) ;
#14562=FACE_OUTER_BOUND ( 'NONE', #10865, .T. ) ;
#14570=ORIENTED_EDGE ( 'NONE', *, *, #14027, .T. ) ;
#14588=VERTEX_POINT ( 'NONE', #17128 ) ;
#14590=VERTEX_POINT ( 'NONE', #13988 ) ;
#14614=ORIENTED_EDGE ( 'NONE', *, *, #15828, .F. ) ;
#14635=DIRECTION ( 'NONE',  ( -1.000000000000000000, -0.000000000000000000, -2.081668171172167774E-16 ) ) ;
#14651=DIRECTION ( 'NONE',  ( -7.709882115452476934E-17, -0.000000000000000000, -1.000000000000000000 ) ) ;
#14681=DIRECTION ( 'NONE',  ( -1.000000000000000000, 0.000000000000000000, -7.304098846218135653E-17 ) ) ;
#14696=VERTEX_POINT ( 'NONE', #6729 ) ;
#14704=DIRECTION ( 'NONE',  ( -7.709882115452476934E-17, -0.000000000000000000, -1.000000000000000000 ) ) ;
#14708=AXIS2_PLACEMENT_3D ( 'NONE', #19326, #5704, #10186 ) ;
#14718=CARTESIAN_POINT ( 'NONE',  ( 50.00000000000000000, 0.000000000000000000, -60.00000000000000000 ) ) ;
#14725=CARTESIAN_POINT ( 'NONE',  ( -37.50000000000002132, -6.000000000000000000, -25.00000000000002132 ) ) ;
#14748=CARTESIAN_POINT ( 'NONE',  ( 44.99999999999998579, 0.000000000000000000, -53.39999999999999147 ) ) ;
#14751=EDGE_CURVE ( 'NONE', #18739, #3513, #370, .T. ) ;
#14791=DIRECTION ( 'NONE',  ( 0.000000000000000000, 1.000000000000000000, 0.000000000000000000 ) ) ;
#14804=EDGE_CURVE ( 'NONE', #8146, #628, #1433, .T. ) ;
#14833=CARTESIAN_POINT ( 'NONE',  ( -32.50000000000002132, -6.000000000000000000, -25.00000000000002132 ) ) ;
#14838=LINE ( 'NONE', #2969, #13934 ) ;
#14844=DIRECTION ( 'NONE',  ( -1.000000000000000000, 0.000000000000000000, -1.541976423090495633E-16 ) ) ;
#14857=LINE ( 'NONE', #10532, #2237 ) ;
#14887=DIRECTION ( 'NONE',  ( 0.000000000000000000, 0.000000000000000000, 1.000000000000000000 ) ) ;
#14890=ADVANCED_FACE ( 'NONE', ( #10164 ), #8339, .F. ) ;
#14915=PLANE ( 'NONE',  #6269 ) ;
#14926=AXIS2_PLACEMENT_3D ( 'NONE', #18168, #4743, #10700 ) ;
#14928=EDGE_LOOP ( 'NONE', ( #19024, #11561, #8986, #1753 ) ) ;
#14947=DIRECTION ( 'NONE',  ( -0.000000000000000000, -1.000000000000000000, -0.000000000000000000 ) ) ;
#14967=VERTEX_POINT ( 'NONE', #12313 ) ;
#14991=EDGE_LOOP ( 'NONE', ( #16246, #16678 ) ) ;
#14995=DIRECTION ( 'NONE',  ( 0.000000000000000000, -1.000000000000000000, 0.000000000000000000 ) ) ;
#14997=VERTEX_POINT ( 'NONE', #4679 ) ;
#14999=EDGE_CURVE ( 'NONE', #8051, #16200, #163, .T. ) ;
#15008=PLANE ( 'NONE',  #8756 ) ;
#15015=SHAPE_DEFINITION_REPRESENTATION ( #3936, #13906 ) ;
#15020=EDGE_CURVE ( 'NONE', #7828, #17265, #18308, .T. ) ;
#15031=VECTOR ( 'NONE', #13914, 1000.000000000000000 ) ;
#15040=VECTOR ( 'NONE', #8722, 1000.000000000000000 ) ;
#15062=FACE_OUTER_BOUND ( 'NONE', #5558, .T. ) ;
#15110=ORIENTED_EDGE ( 'NONE', *, *, #5891, .T. ) ;
#15115=LINE ( 'NONE', #16282, #11295 ) ;
#15136=CARTESIAN_POINT ( 'NONE',  ( -37.50000000000002132, -6.000000000000000000, 24.99999999999998224 ) ) ;
#15155=DIRECTION ( 'NONE',  ( -7.709882115452476934E-17, -0.000000000000000000, -1.000000000000000000 ) ) ;
#15182=DIRECTION ( 'NONE',  ( 1.000000000000000000, 0.000000000000000000, 2.973811673103096679E-16 ) ) ;
#15185=VERTEX_POINT ( 'NONE', #17217 ) ;
#15193=ORIENTED_EDGE ( 'NONE', *, *, #5989, .F. ) ;
#15196=( LENGTH_UNIT ( ) NAMED_UNIT ( * ) SI_UNIT ( .MILLI., .METRE. ) );
#15204=CARTESIAN_POINT ( 'NONE',  ( -45.00000000000000000, 3.000000000000000000, 53.39999999999999147 ) ) ;
#15208=ORIENTED_EDGE ( 'NONE', *, *, #1859, .T. ) ;
#15215=DIRECTION ( 'NONE',  ( -7.709882115452476934E-17, -0.000000000000000000, -1.000000000000000000 ) ) ;
#15221=ORIENTED_EDGE ( 'NONE', *, *, #14193, .F. ) ;
#15260=EDGE_CURVE ( 'NONE', #18667, #13252, #17309, .T. ) ;
#15271=DIRECTION ( 'NONE',  ( -0.000000000000000000, 1.000000000000000000, -0.000000000000000000 ) ) ;
#15285=ORIENTED_EDGE ( 'NONE', *, *, #8335, .T. ) ;
#15302=DIRECTION ( 'NONE',  ( -1.000000000000000000, 0.000000000000000000, -7.304098846218135653E-17 ) ) ;
#15342=LINE ( 'NONE', #16918, #393 ) ;
#15368=CARTESIAN_POINT ( 'NONE',  ( -37.50000000000002132, -6.000000000000000000, -25.00000000000002132 ) ) ;
#15376=DIRECTION ( 'NONE',  ( -0.000000000000000000, -1.000000000000000000, -0.000000000000000000 ) ) ;
#15377=CIRCLE ( 'NONE', #10015, 1.599999999999997202 ) ;
#15384=DIRECTION ( 'NONE',  ( -1.000000000000000000, 0.000000000000000000, 0.000000000000000000 ) ) ;
#15401=CARTESIAN_POINT ( 'NONE',  ( -25.00000000000001421, -6.000000000000000000, 42.49999999999997868 ) ) ;
#15408=FACE_OUTER_BOUND ( 'NONE', #10879, .T. ) ;
#15418=VECTOR ( 'NONE', #9172, 1000.000000000000000 ) ;
#15447=CARTESIAN_POINT ( 'NONE',  ( 44.99999999999997158, -1.285879139104706187E-16, 53.40000000000000568 ) ) ;
#15451=CARTESIAN_POINT ( 'NONE',  ( -14.99999999999999645, 73.00000000000001421, 26.99999999999997868 ) ) ;
#15452=CARTESIAN_POINT ( 'NONE',  ( 37.49999999999999289, 0.000000000000000000, -25.00000000000001421 ) ) ;
#15467=ORIENTED_EDGE ( 'NONE', *, *, #14027, .F. ) ;
#15470=CARTESIAN_POINT ( 'NONE',  ( -44.99999999999998579, -1.285879139104706187E-16, -55.00000000000000000 ) ) ;
#15472=CARTESIAN_POINT ( 'NONE',  ( -25.00000000000000711, -6.000000000000000000, -47.50000000000002132 ) ) ;
#15473=EDGE_CURVE ( 'NONE', #16010, #12630, #8958, .T. ) ;
#15474=CARTESIAN_POINT ( 'NONE',  ( -37.50000000000002132, 107.3545527679194436, 24.99999999999998224 ) ) ;
#15477=EDGE_CURVE ( 'NONE', #428, #17877, #16145, .T. ) ;
#15497=DIRECTION ( 'NONE',  ( -0.000000000000000000, -1.000000000000000000, -0.000000000000000000 ) ) ;
#15502=CARTESIAN_POINT ( 'NONE',  ( 34.99999999999999289, -6.000000000000000000, 47.49999999999997868 ) ) ;
#15508=ORIENTED_EDGE ( 'NONE', *, *, #4849, .T. ) ;
#15520=AXIS2_PLACEMENT_3D ( 'NONE', #14517, #4231, #11667 ) ;
#15527=FACE_BOUND ( 'NONE', #12241, .T. ) ;
#15529=( NAMED_UNIT ( * ) SI_UNIT ( $, .STERADIAN. ) SOLID_ANGLE_UNIT ( ) );
#15570=AXIS2_PLACEMENT_3D ( 'NONE', #1374, #11651, #3033 ) ;
#15616=ADVANCED_FACE ( 'NONE', ( #6224 ), #10911, .T. ) ;
#15636=EDGE_CURVE ( 'NONE', #10068, #14997, #12295, .T. ) ;
#15641=VECTOR ( 'NONE', #11140, 1000.000000000000000 ) ;
#15654=AXIS2_PLACEMENT_3D ( 'NONE', #13131, #17653, #4228 ) ;
#15663=FACE_OUTER_BOUND ( 'NONE', #4200, .T. ) ;
#15665=VECTOR ( 'NONE', #15182, 1000.000000000000000 ) ;
#15676=ORIENTED_EDGE ( 'NONE', *, *, #7869, .F. ) ;
#15685=AXIS2_PLACEMENT_3D ( 'NONE', #12528, #12333, #18428 ) ;
#15691=DIRECTION ( 'NONE',  ( -1.000000000000000000, 0.000000000000000000, -9.251858538542970348E-17 ) ) ;
#15704=LINE ( 'NONE', #6780, #3024 ) ;
#15707=VECTOR ( 'NONE', #1637, 1000.000000000000000 ) ;
#15713=DIRECTION ( 'NONE',  ( 1.000000000000000000, 0.000000000000000000, 0.000000000000000000 ) ) ;
#15721=EDGE_CURVE ( 'NONE', #10544, #1168, #7790, .T. ) ;
#15725=CARTESIAN_POINT ( 'NONE',  ( 32.49999999999998579, -6.000000000000000000, 24.99999999999998224 ) ) ;
#15774=FACE_BOUND ( 'NONE', #14991, .T. ) ;
#15783=PRODUCT_DEFINITION ( 'UNKNOWN', '', #5174, #9431 ) ;
#15804=ORIENTED_EDGE ( 'NONE', *, *, #616, .T. ) ;
#15828=EDGE_CURVE ( 'NONE', #5969, #10544, #3759, .T. ) ;
#15845=ORIENTED_EDGE ( 'NONE', *, *, #14999, .T. ) ;
#15849=CARTESIAN_POINT ( 'NONE',  ( -50.00000000000002132, 3.000000000000000000, -60.00000000000002132 ) ) ;
#15855=VECTOR ( 'NONE', #4242, 1000.000000000000000 ) ;
#15857=PLANE ( 'NONE',  #8333 ) ;
#15859=VERTEX_POINT ( 'NONE', #11380 ) ;
#15870=MECHANICAL_DESIGN_GEOMETRIC_PRESENTATION_REPRESENTATION('',(#12096),#7739);
#15879=EDGE_CURVE ( 'NONE', #19310, #9095, #6483, .T. ) ;
#15886=DIRECTION ( 'NONE',  ( -0.000000000000000000, 1.000000000000000000, -0.000000000000000000 ) ) ;
#15893=EDGE_LOOP ( 'NONE', ( #10209, #18087, #17716, #13171 ) ) ;
#15903=CARTESIAN_POINT ( 'NONE',  ( 49.99999999999998579, 0.000000000000000000, 59.99999999999997868 ) ) ;
#15905=CARTESIAN_POINT ( 'NONE',  ( 24.99999999999998579, -6.000000000000000000, 42.49999999999997868 ) ) ;
#15912=VECTOR ( 'NONE', #4183, 1000.000000000000000 ) ;
#15921=VECTOR ( 'NONE', #16525, 1000.000000000000000 ) ;
#15924=DIRECTION ( 'NONE',  ( 0.000000000000000000, 0.000000000000000000, -1.000000000000000000 ) ) ;
#15933=VECTOR ( 'NONE', #19276, 1000.000000000000000 ) ;
#16000=DIRECTION ( 'NONE',  ( -1.000000000000000000, 0.000000000000000000, -9.251858538542970348E-17 ) ) ;
#16003=CARTESIAN_POINT ( 'NONE',  ( 24.99999999999999289, -6.000000000000000000, -42.49999999999999289 ) ) ;
#16004=CIRCLE ( 'NONE', #7550, 2.999999999999999112 ) ;
#16008=CLOSED_SHELL ( 'NONE', ( #785, #8781, #10224, #16708, #6622, #5879, #14037, #1750, #18644, #19222, #16297, #14890, #17998, #16817, #13955, #9540, #7012, #14527, #12520, #2723, #3986, #17625, #2633, #11054, #15616, #12402, #19132, #1903, #10894, #14033, #8951, #10398, #6280, #12594, #18285, #14024, #17987, #2310, #5098, #17782, #12496, #7990, #13659, #4262, #6039, #5096, #378, #6907 ) ) ;
#16010=VERTEX_POINT ( 'NONE', #600 ) ;
#16040=CARTESIAN_POINT ( 'NONE',  ( 14.99999999999998579, 3.000000000000000000, 20.99999999999997513 ) ) ;
#16051=EDGE_LOOP ( 'NONE', ( #8367, #8406, #1473, #2643, #7745, #9799 ) ) ;
#16057=ORIENTED_EDGE ( 'NONE', *, *, #11323, .F. ) ;
#16068=CARTESIAN_POINT ( 'NONE',  ( -44.99999999999998579, -1.285879139104706187E-16, -55.00000000000000000 ) ) ;
#16079=ORIENTED_EDGE ( 'NONE', *, *, #17798, .F. ) ;
#16128=VECTOR ( 'NONE', #7338, 1000.000000000000000 ) ;
#16141=ORIENTED_EDGE ( 'NONE', *, *, #1859, .F. ) ;
#16143=VECTOR ( 'NONE', #12624, 1000.000000000000000 ) ;
#16145=CIRCLE ( 'NONE', #2087, 2.999999999999999112 ) ;
#16146=PLANE ( 'NONE',  #16933 ) ;
#16156=ORIENTED_EDGE ( 'NONE', *, *, #12530, .F. ) ;
#16158=CARTESIAN_POINT ( 'NONE',  ( -35.00000000000002132, -6.000000000000000000, -47.50000000000002132 ) ) ;
#16175=AXIS2_PLACEMENT_3D ( 'NONE', #6566, #8043, #3234 ) ;
#16181=PLANE ( 'NONE',  #14708 ) ;
#16200=VERTEX_POINT ( 'NONE', #6396 ) ;
#16211=FACE_OUTER_BOUND ( 'NONE', #6569, .T. ) ;
#16226=CARTESIAN_POINT ( 'NONE',  ( 14.99999999999998579, 73.00000000000001421, 26.99999999999997158 ) ) ;
#16239=ORIENTED_EDGE ( 'NONE', *, *, #14751, .T. ) ;
#16246=ORIENTED_EDGE ( 'NONE', *, *, #821, .F. ) ;
#16249=LINE ( 'NONE', #18649, #18529 ) ;
#16252=DIRECTION ( 'NONE',  ( -7.709882115452476934E-17, -0.000000000000000000, -1.000000000000000000 ) ) ;
#16272=FACE_OUTER_BOUND ( 'NONE', #1699, .T. ) ;
#16280=DIRECTION ( 'NONE',  ( -0.000000000000000000, -1.000000000000000000, -0.000000000000000000 ) ) ;
#16282=CARTESIAN_POINT ( 'NONE',  ( 32.50000000000000000, -6.000000000000000000, -45.00000000000000000 ) ) ;
#16297=ADVANCED_FACE ( 'NONE', ( #12360 ), #10782, .F. ) ;
#16301=VECTOR ( 'NONE', #13651, 1000.000000000000000 ) ;
#16305=EDGE_CURVE ( 'NONE', #2520, #18340, #315, .T. ) ;
#16353=LINE ( 'NONE', #7826, #5385 ) ;
#16377=CYLINDRICAL_SURFACE ( 'NONE', #11230, 2.999999999999999112 ) ;
#16378=CARTESIAN_POINT ( 'NONE',  ( -50.00000000000002132, 3.000000000000000000, -60.00000000000002132 ) ) ;
#16379=EDGE_LOOP ( 'NONE', ( #865, #1472, #6911, #6583 ) ) ;
#16394=DIRECTION ( 'NONE',  ( 0.000000000000000000, -1.000000000000000000, 0.000000000000000000 ) ) ;
#16432=CARTESIAN_POINT ( 'NONE',  ( -32.50000000000002132, 0.000000000000000000, 24.99999999999998224 ) ) ;
#16436=ORIENTED_EDGE ( 'NONE', *, *, #6683, .F. ) ;
#16449=VERTEX_POINT ( 'NONE', #18209 ) ;
#16463=DIRECTION ( 'NONE',  ( 0.000000000000000000, 0.000000000000000000, -1.000000000000000000 ) ) ;
#16466=VERTEX_POINT ( 'NONE', #15452 ) ;
#16472=LINE ( 'NONE', #9015, #18768 ) ;
#16486=LINE ( 'NONE', #2752, #18339 ) ;
#16493=VECTOR ( 'NONE', #5132, 1000.000000000000000 ) ;
#16502=LINE ( 'NONE', #19247, #10321 ) ;
#16505=ORIENTED_EDGE ( 'NONE', *, *, #11494, .T. ) ;
#16525=DIRECTION ( 'NONE',  ( -7.709882115452476934E-17, -0.000000000000000000, -1.000000000000000000 ) ) ;
#16541=PLANE ( 'NONE',  #17700 ) ;
#16554=DIRECTION ( 'NONE',  ( 0.000000000000000000, -1.000000000000000000, 0.000000000000000000 ) ) ;
#16566=CARTESIAN_POINT ( 'NONE',  ( -14.99999999999999645, 73.00000000000001421, 23.99999999999997868 ) ) ;
#16579=ORIENTED_EDGE ( 'NONE', *, *, #303, .T. ) ;
#16607=DIRECTION ( 'NONE',  ( -7.304098846218135653E-17, 0.000000000000000000, 1.000000000000000000 ) ) ;
#16639=DIRECTION ( 'NONE',  ( 1.000000000000000000, 0.000000000000000000, -7.709882115452476934E-17 ) ) ;
#16641=CARTESIAN_POINT ( 'NONE',  ( -50.00000000000001421, 0.000000000000000000, 59.99999999999997868 ) ) ;
#16653=DIRECTION ( 'NONE',  ( -0.000000000000000000, -1.000000000000000000, -0.000000000000000000 ) ) ;
#16676=DIRECTION ( 'NONE',  ( 9.251858538542970348E-17, 0.000000000000000000, -1.000000000000000000 ) ) ;
#16678=ORIENTED_EDGE ( 'NONE', *, *, #6802, .F. ) ;
#16690=DIRECTION ( 'NONE',  ( -0.000000000000000000, -1.000000000000000000, -0.000000000000000000 ) ) ;
#16701=CARTESIAN_POINT ( 'NONE',  ( -45.00000000000000000, 3.000000000000000000, 56.59999999999998010 ) ) ;
#16708=ADVANCED_FACE ( 'NONE', ( #1119 ), #8288, .F. ) ;
#16776=PLANE ( 'NONE',  #1895 ) ;
#16778=CYLINDRICAL_SURFACE ( 'NONE', #1298, 1.599999999999997202 ) ;
#16789=VERTEX_POINT ( 'NONE', #19356 ) ;
#16817=ADVANCED_FACE ( 'NONE', ( #16211 ), #1322, .F. ) ;
#16850=LINE ( 'NONE', #7934, #17571 ) ;
#16872=VERTEX_POINT ( 'NONE', #9446 ) ;
#16882=CYLINDRICAL_SURFACE ( 'NONE', #10642, 1.599999999999997202 ) ;
#16889=ORIENTED_EDGE ( 'NONE', *, *, #1242, .T. ) ;
#16902=CARTESIAN_POINT ( 'NONE',  ( 0.000000000000000000, 3.000000000000000000, 0.000000000000000000 ) ) ;
#16909=ORIENTED_EDGE ( 'NONE', *, *, #1469, .F. ) ;
#16918=CARTESIAN_POINT ( 'NONE',  ( -45.00000000000000000, 0.000000000000000000, 56.59999999999998010 ) ) ;
#16927=CARTESIAN_POINT ( 'NONE',  ( 44.99999999999998579, 3.000000000000000000, -54.99999999999998579 ) ) ;
#16933=AXIS2_PLACEMENT_3D ( 'NONE', #7226, #172, #10351 ) ;
#16938=MANIFOLD_SOLID_BREP ( 'Cut-Extrude-Thin1', #16008 ) ;
#16952=AXIS2_PLACEMENT_3D ( 'NONE', #15474, #18330, #2042 ) ;
#16965=( LENGTH_UNIT ( ) NAMED_UNIT ( * ) SI_UNIT ( .MILLI., .METRE. ) );
#16995=ORIENTED_EDGE ( 'NONE', *, *, #9041, .T. ) ;
#16998=LINE ( 'NONE', #6409, #10009 ) ;
#17042=ORIENTED_EDGE ( 'NONE', *, *, #18009, .T. ) ;
#17048=CARTESIAN_POINT ( 'NONE',  ( 32.49999999999998579, -6.000000000000000000, 42.49999999999997868 ) ) ;
#17049=DIRECTION ( 'NONE',  ( -0.000000000000000000, 0.000000000000000000, -1.000000000000000000 ) ) ;
#17069=CARTESIAN_POINT ( 'NONE',  ( -37.50000000000002132, -6.000000000000000000, 44.99999999999997868 ) ) ;
#17099=DIRECTION ( 'NONE',  ( 1.000000000000000000, 0.000000000000000000, 9.251858538542970348E-17 ) ) ;
#17104=ORIENTED_EDGE ( 'NONE', *, *, #303, .F. ) ;
#17115=AXIS2_PLACEMENT_3D ( 'NONE', #15502, #1686, #7768 ) ;
#17117=DIRECTION ( 'NONE',  ( 0.000000000000000000, -1.000000000000000000, 0.000000000000000000 ) ) ;
#17128=CARTESIAN_POINT ( 'NONE',  ( -25.00000000000001421, -6.000000000000000000, 42.49999999999997868 ) ) ;
#17136=CARTESIAN_POINT ( 'NONE',  ( 49.99999999999998579, 3.000000000000000000, 59.99999999999997868 ) ) ;
#17142=ORIENTED_EDGE ( 'NONE', *, *, #11190, .T. ) ;
#17147=EDGE_LOOP ( 'NONE', ( #7429, #12718, #10081, #1749 ) ) ;
#17196=CARTESIAN_POINT ( 'NONE',  ( 37.49999999999999289, -6.000000000000000000, 47.49999999999997868 ) ) ;
#17217=CARTESIAN_POINT ( 'NONE',  ( 37.49999999999999289, 0.000000000000000000, 24.99999999999998579 ) ) ;
#17218=EDGE_LOOP ( 'NONE', ( #6970, #6509, #13694, #7446 ) ) ;
#17235=VECTOR ( 'NONE', #13016, 1000.000000000000000 ) ;
#17237=ORIENTED_EDGE ( 'NONE', *, *, #12367, .F. ) ;
#17240=VERTEX_POINT ( 'NONE', #19236 ) ;
#17261=CARTESIAN_POINT ( 'NONE',  ( 14.99999999999998579, 73.00000000000001421, 26.99999999999997158 ) ) ;
#17265=VERTEX_POINT ( 'NONE', #7669 ) ;
#17277=VECTOR ( 'NONE', #739, 1000.000000000000000 ) ;
#17309=LINE ( 'NONE', #17397, #8336 ) ;
#17329=EDGE_LOOP ( 'NONE', ( #4613, #4290, #17928, #8713, #1556, #18507 ) ) ;
#17345=CARTESIAN_POINT ( 'NONE',  ( 44.99999999999998579, -1.285879139104706187E-16, -56.59999999999998010 ) ) ;
#17352=ORIENTED_EDGE ( 'NONE', *, *, #138, .T. ) ;
#17357=EDGE_CURVE ( 'NONE', #2050, #2908, #4835, .T. ) ;
#17377=AXIS2_PLACEMENT_3D ( 'NONE', #9812, #5601, #5707 ) ;
#17397=CARTESIAN_POINT ( 'NONE',  ( -25.00000000000001421, 107.3545527679194436, 47.49999999999997868 ) ) ;
#17420=EDGE_LOOP ( 'NONE', ( #5599, #2923 ) ) ;
#17438=CARTESIAN_POINT ( 'NONE',  ( 44.99999999999998579, 3.000000000000000000, -56.59999999999998010 ) ) ;
#17443=DIRECTION ( 'NONE',  ( -0.000000000000000000, -1.000000000000000000, -0.000000000000000000 ) ) ;
#17459=CARTESIAN_POINT ( 'NONE',  ( 37.50000000000000711, -6.000000000000000000, -45.00000000000000000 ) ) ;
#17465=ORIENTED_EDGE ( 'NONE', *, *, #18972, .F. ) ;
#17487=AXIS2_PLACEMENT_3D ( 'NONE', #3387, #10730, #6433 ) ;
#17529=AXIS2_PLACEMENT_3D ( 'NONE', #12451, #18448, #5018 ) ;
#17541=ORIENTED_EDGE ( 'NONE', *, *, #5368, .T. ) ;
#17571=VECTOR ( 'NONE', #2230, 1000.000000000000000 ) ;
#17606=LINE ( 'NONE', #15849, #15912 ) ;
#17625=ADVANCED_FACE ( 'NONE', ( #13309 ), #1565, .F. ) ;
#17641=FACE_OUTER_BOUND ( 'NONE', #12783, .T. ) ;
#17648=FACE_OUTER_BOUND ( 'NONE', #13395, .T. ) ;
#17653=DIRECTION ( 'NONE',  ( 0.000000000000000000, 1.000000000000000000, -0.000000000000000000 ) ) ;
#17661=AXIS2_PLACEMENT_3D ( 'NONE', #43, #14844, #19259 ) ;
#17676=DIRECTION ( 'NONE',  ( -0.000000000000000000, 0.000000000000000000, -1.000000000000000000 ) ) ;
#17700=AXIS2_PLACEMENT_3D ( 'NONE', #13289, #19387, #5862 ) ;
#17711=VECTOR ( 'NONE', #13707, 1000.000000000000000 ) ;
#17716=ORIENTED_EDGE ( 'NONE', *, *, #5368, .F. ) ;
#17728=LINE ( 'NONE', #10561, #904 ) ;
#17734=CARTESIAN_POINT ( 'NONE',  ( -37.50000000000002132, -6.000000000000000000, 44.99999999999997868 ) ) ;
#17735=CARTESIAN_POINT ( 'NONE',  ( -50.00000000000001421, 3.000000000000000000, 59.99999999999997868 ) ) ;
#17753=EDGE_CURVE ( 'NONE', #4517, #19239, #8706, .T. ) ;
#17776=LINE ( 'NONE', #8852, #10936 ) ;
#17782=ADVANCED_FACE ( 'NONE', ( #4612 ), #12240, .T. ) ;
#17785=EDGE_CURVE ( 'NONE', #16789, #18739, #10957, .T. ) ;
#17790=ORIENTED_EDGE ( 'NONE', *, *, #423, .F. ) ;
#17798=EDGE_CURVE ( 'NONE', #8432, #14106, #1760, .T. ) ;
#17808=DIRECTION ( 'NONE',  ( 0.000000000000000000, 0.000000000000000000, 1.000000000000000000 ) ) ;
#17813=VECTOR ( 'NONE', #8331, 1000.000000000000000 ) ;
#17820=AXIS2_PLACEMENT_3D ( 'NONE', #12646, #2350, #18643 ) ;
#17824=EDGE_CURVE ( 'NONE', #15185, #1168, #9202, .T. ) ;
#17826=DIRECTION ( 'NONE',  ( -7.304098846218135653E-17, 0.000000000000000000, 1.000000000000000000 ) ) ;
#17831=AXIS2_PLACEMENT_3D ( 'NONE', #8049, #16676, #18145 ) ;
#17836=VECTOR ( 'NONE', #12554, 1000.000000000000000 ) ;
#17849=CARTESIAN_POINT ( 'NONE',  ( 14.99999999999998579, 73.00000000000001421, 23.99999999999997158 ) ) ;
#17877=VERTEX_POINT ( 'NONE', #284 ) ;
#17883=DIRECTION ( 'NONE',  ( -0.000000000000000000, -1.000000000000000000, -0.000000000000000000 ) ) ;
#17909=CARTESIAN_POINT ( 'NONE',  ( -35.00000000000002132, -0.000000000000000000, -42.50000000000001421 ) ) ;
#17911=AXIS2_PLACEMENT_3D ( 'NONE', #10704, #14010, #11343 ) ;
#17921=VERTEX_POINT ( 'NONE', #12900 ) ;
#17926=CARTESIAN_POINT ( 'NONE',  ( -14.99999999999999645, 73.00000000000001421, 20.99999999999998224 ) ) ;
#17928=ORIENTED_EDGE ( 'NONE', *, *, #10831, .T. ) ;
#17941=ORIENTED_EDGE ( 'NONE', *, *, #19117, .F. ) ;
#17948=LINE ( 'NONE', #7351, #11869 ) ;
#17974=ORIENTED_EDGE ( 'NONE', *, *, #18977, .F. ) ;
#17976=CARTESIAN_POINT ( 'NONE',  ( 24.99999999999998579, 107.3545527679194436, 47.49999999999997868 ) ) ;
#17987=ADVANCED_FACE ( 'NONE', ( #18710 ), #3890, .T. ) ;
#17998=ADVANCED_FACE ( 'NONE', ( #9859 ), #15857, .F. ) ;
#18009=EDGE_CURVE ( 'NONE', #9993, #17921, #14372, .T. ) ;
#18027=DIRECTION ( 'NONE',  ( 7.304098846218135653E-17, 0.000000000000000000, -1.000000000000000000 ) ) ;
#18029=ORIENTED_EDGE ( 'NONE', *, *, #2116, .F. ) ;
#18037=VECTOR ( 'NONE', #4310, 1000.000000000000000 ) ;
#18041=ORIENTED_EDGE ( 'NONE', *, *, #4258, .F. ) ;
#18067=CIRCLE ( 'NONE', #19319, 1.599999999999997202 ) ;
#18087=ORIENTED_EDGE ( 'NONE', *, *, #4258, .T. ) ;
#18098=CARTESIAN_POINT ( 'NONE',  ( 37.50000000000000711, 0.000000000000000000, -45.00000000000000000 ) ) ;
#18102=DIRECTION ( 'NONE',  ( -7.709882115452476934E-17, 0.000000000000000000, -1.000000000000000000 ) ) ;
#18106=DIRECTION ( 'NONE',  ( -7.709882115452476934E-17, 0.000000000000000000, -1.000000000000000000 ) ) ;
#18115=ORIENTED_EDGE ( 'NONE', *, *, #8565, .F. ) ;
#18133=ORIENTED_EDGE ( 'NONE', *, *, #2860, .T. ) ;
#18138=( NAMED_UNIT ( * ) PLANE_ANGLE_UNIT ( ) SI_UNIT ( $, .RADIAN. ) );
#18145=DIRECTION ( 'NONE',  ( -1.000000000000000000, 0.000000000000000000, -9.251858538542970348E-17 ) ) ;
#18157=LINE ( 'NONE', #10689, #12245 ) ;
#18161=LINE ( 'NONE', #10692, #22 ) ;
#18168=CARTESIAN_POINT ( 'NONE',  ( -44.99999999999998579, 3.000000000000000000, -55.00000000000000000 ) ) ;
#18169=ORIENTED_EDGE ( 'NONE', *, *, #4354, .T. ) ;
#18186=FILL_AREA_STYLE_COLOUR ( '', #6709 ) ;
#18197=VECTOR ( 'NONE', #15384, 1000.000000000000000 ) ;
#18205=VECTOR ( 'NONE', #7134, 1000.000000000000000 ) ;
#18209=CARTESIAN_POINT ( 'NONE',  ( 24.99999999999999289, -6.000000000000000000, -42.49999999999999289 ) ) ;
#18222=CIRCLE ( 'NONE', #18846, 2.999999999999999112 ) ;
#18248=AXIS2_PLACEMENT_3D ( 'NONE', #19300, #14791, #14887 ) ;
#18257=VERTEX_POINT ( 'NONE', #18990 ) ;
#18285=ADVANCED_FACE ( 'NONE', ( #2104 ), #5241, .F. ) ;
#18308=LINE ( 'NONE', #3393, #18037 ) ;
#18322=ORIENTED_EDGE ( 'NONE', *, *, #6184, .T. ) ;
#18326=AXIS2_PLACEMENT_3D ( 'NONE', #17976, #13254, #8853 ) ;
#18327=ORIENTED_EDGE ( 'NONE', *, *, #9041, .F. ) ;
#18330=DIRECTION ( 'NONE',  ( 9.251858538542970348E-17, 0.000000000000000000, -1.000000000000000000 ) ) ;
#18339=VECTOR ( 'NONE', #6001, 1000.000000000000000 ) ;
#18340=VERTEX_POINT ( 'NONE', #16641 ) ;
#18345=VERTEX_POINT ( 'NONE', #17196 ) ;
#18421=ORIENTED_EDGE ( 'NONE', *, *, #1921, .T. ) ;
#18424=CARTESIAN_POINT ( 'NONE',  ( -50.00000000000001421, 3.000000000000000000, 59.99999999999997868 ) ) ;
#18428=DIRECTION ( 'NONE',  ( -7.709882115452476934E-17, 0.000000000000000000, -1.000000000000000000 ) ) ;
#18440=PLANE ( 'NONE',  #17831 ) ;
#18447=CARTESIAN_POINT ( 'NONE',  ( -37.50000000000002132, 0.000000000000000000, -25.00000000000002132 ) ) ;
#18448=DIRECTION ( 'NONE',  ( 0.000000000000000000, -1.000000000000000000, 0.000000000000000000 ) ) ;
#18458=ORIENTED_EDGE ( 'NONE', *, *, #654, .T. ) ;
#18480=CARTESIAN_POINT ( 'NONE',  ( -44.99999999999998579, 3.000000000000000000, -55.00000000000000000 ) ) ;
#18491=DIRECTION ( 'NONE',  ( -0.000000000000000000, -1.000000000000000000, -0.000000000000000000 ) ) ;
#18507=ORIENTED_EDGE ( 'NONE', *, *, #17753, .F. ) ;
#18519=EDGE_LOOP ( 'NONE', ( #13263, #13648, #18421, #9678 ) ) ;
#18529=VECTOR ( 'NONE', #11940, 1000.000000000000000 ) ;
#18557=EDGE_CURVE ( 'NONE', #6502, #10761, #19040, .T. ) ;
#18559=CARTESIAN_POINT ( 'NONE',  ( -44.99999999999998579, 3.000000000000000000, -56.59999999999999432 ) ) ;
#18598=VERTEX_POINT ( 'NONE', #18947 ) ;
#18613=DIRECTION ( 'NONE',  ( -0.000000000000000000, 1.000000000000000000, -0.000000000000000000 ) ) ;
#18630=FACE_OUTER_BOUND ( 'NONE', #5884, .T. ) ;
#18638=EDGE_CURVE ( 'NONE', #15185, #5969, #223, .T. ) ;
#18643=DIRECTION ( 'NONE',  ( 0.000000000000000000, 0.000000000000000000, -1.000000000000000000 ) ) ;
#18644=ADVANCED_FACE ( 'NONE', ( #6208 ), #6010, .T. ) ;
#18649=CARTESIAN_POINT ( 'NONE',  ( -37.50000000000002842, -6.000000000000000000, -47.50000000000002132 ) ) ;
#18656=CARTESIAN_POINT ( 'NONE',  ( -45.00000000000000000, 3.000000000000000000, 54.99999999999998579 ) ) ;
#18657=ORIENTED_EDGE ( 'NONE', *, *, #7350, .T. ) ;
#18667=VERTEX_POINT ( 'NONE', #10496 ) ;
#18687=DIRECTION ( 'NONE',  ( -0.000000000000000000, -1.000000000000000000, -0.000000000000000000 ) ) ;
#18710=FACE_OUTER_BOUND ( 'NONE', #18519, .T. ) ;
#18735=CARTESIAN_POINT ( 'NONE',  ( -50.00000000000002132, 3.000000000000000000, -60.00000000000002132 ) ) ;
#18739=VERTEX_POINT ( 'NONE', #14725 ) ;
#18753=FACE_OUTER_BOUND ( 'NONE', #13343, .T. ) ;
#18768=VECTOR ( 'NONE', #5887, 1000.000000000000000 ) ;
#18794=CARTESIAN_POINT ( 'NONE',  ( -25.00000000000001421, 0.000000000000000000, 47.49999999999997868 ) ) ;
#18802=ORIENTED_EDGE ( 'NONE', *, *, #16305, .T. ) ;
#18804=EDGE_LOOP ( 'NONE', ( #11840, #16156, #3350, #1670 ) ) ;
#18812=FACE_BOUND ( 'NONE', #2724, .T. ) ;
#18835=VECTOR ( 'NONE', #497, 1000.000000000000000 ) ;
#18841=APPLICATION_CONTEXT ( 'automotive_design' ) ;
#18846=AXIS2_PLACEMENT_3D ( 'NONE', #1729, #10834, #255 ) ;
#18847=LINE ( 'NONE', #8539, #13112 ) ;
#18850=FACE_OUTER_BOUND ( 'NONE', #12834, .T. ) ;
#18880=EDGE_CURVE ( 'NONE', #15859, #10068, #14034, .T. ) ;
#18921=ORIENTED_EDGE ( 'NONE', *, *, #1811, .F. ) ;
#18924=DIRECTION ( 'NONE',  ( -7.709882115452476934E-17, -0.000000000000000000, -1.000000000000000000 ) ) ;
#18932=EDGE_LOOP ( 'NONE', ( #1240, #3995 ) ) ;
#18947=CARTESIAN_POINT ( 'NONE',  ( -45.00000000000000000, -1.285879139104706187E-16, 53.39999999999999147 ) ) ;
#18970=DIRECTION ( 'NONE',  ( 0.000000000000000000, 1.000000000000000000, -0.000000000000000000 ) ) ;
#18972=EDGE_CURVE ( 'NONE', #9095, #19310, #13013, .T. ) ;
#18976=CARTESIAN_POINT ( 'NONE',  ( -32.50000000000001421, 0.000000000000000000, 44.99999999999997868 ) ) ;
#18977=EDGE_CURVE ( 'NONE', #14696, #17240, #5406, .T. ) ;
#18990=CARTESIAN_POINT ( 'NONE',  ( 49.99999999999998579, 3.000000000000000000, 59.99999999999997868 ) ) ;
#18997=ORIENTED_EDGE ( 'NONE', *, *, #11373, .F. ) ;
#19024=ORIENTED_EDGE ( 'NONE', *, *, #12367, .T. ) ;
#19040=LINE ( 'NONE', #15905, #1775 ) ;
#19065=EDGE_CURVE ( 'NONE', #2050, #11844, #15704, .T. ) ;
#19075=CARTESIAN_POINT ( 'NONE',  ( -35.00000000000002132, -6.000000000000000000, -42.50000000000001421 ) ) ;
#19091=VERTEX_POINT ( 'NONE', #14407 ) ;
#19106=CARTESIAN_POINT ( 'NONE',  ( 34.99999999999999289, -6.000000000000000000, 47.49999999999997868 ) ) ;
#19117=EDGE_CURVE ( 'NONE', #3455, #2845, #18067, .T. ) ;
#19130=FACE_OUTER_BOUND ( 'NONE', #6188, .T. ) ;
#19132=ADVANCED_FACE ( 'NONE', ( #2272 ), #14226, .T. ) ;
#19142=CIRCLE ( 'NONE', #10682, 1.599999999999997202 ) ;
#19165=AXIS2_PLACEMENT_3D ( 'NONE', #5449, #2595, #13267 ) ;
#19197=VERTEX_POINT ( 'NONE', #11550 ) ;
#19199=CARTESIAN_POINT ( 'NONE',  ( 14.99999999999998579, 3.000000000000000000, 23.99999999999997158 ) ) ;
#19201=EDGE_LOOP ( 'NONE', ( #14042, #15508, #17790, #13886 ) ) ;
#19202=DIRECTION ( 'NONE',  ( -1.000000000000000000, 0.000000000000000000, 0.000000000000000000 ) ) ;
#19222=ADVANCED_FACE ( 'NONE', ( #17641 ), #10379, .T. ) ;
#19236=CARTESIAN_POINT ( 'NONE',  ( -32.50000000000002132, -0.000000000000000000, -42.50000000000001421 ) ) ;
#19239=VERTEX_POINT ( 'NONE', #10571 ) ;
#19242=EDGE_CURVE ( 'NONE', #717, #2416, #10859, .T. ) ;
#19247=CARTESIAN_POINT ( 'NONE',  ( -35.00000000000002132, -6.000000000000000000, -47.50000000000002132 ) ) ;
#19251=ORIENTED_EDGE ( 'NONE', *, *, #14804, .F. ) ;
#19259=DIRECTION ( 'NONE',  ( -1.541976423090495633E-16, 0.000000000000000000, 1.000000000000000000 ) ) ;
#19276=DIRECTION ( 'NONE',  ( 1.000000000000000000, 0.000000000000000000, 2.973811673103096679E-16 ) ) ;
#19298=ORIENTED_EDGE ( 'NONE', *, *, #7350, .F. ) ;
#19300=CARTESIAN_POINT ( 'NONE',  ( -14.99999999999999645, 3.000000000000000000, 23.99999999999997868 ) ) ;
#19310=VERTEX_POINT ( 'NONE', #12046 ) ;
#19319=AXIS2_PLACEMENT_3D ( 'NONE', #18656, #5221, #6961 ) ;
#19326=CARTESIAN_POINT ( 'NONE',  ( 14.99999999999998579, 73.00000000000001421, 23.99999999999997158 ) ) ;
#19335=EDGE_CURVE ( 'NONE', #14997, #19197, #13412, .T. ) ;
#19337=EDGE_CURVE ( 'NONE', #13561, #8432, #8977, .T. ) ;
#19347=CARTESIAN_POINT ( 'NONE',  ( 34.99999999999999289, 0.000000000000000000, 47.49999999999997868 ) ) ;
#19351=DIRECTION ( 'NONE',  ( 1.000000000000000000, 0.000000000000000000, 2.973811673103096679E-16 ) ) ;
#19356=CARTESIAN_POINT ( 'NONE',  ( -37.50000000000002132, 0.000000000000000000, -25.00000000000002132 ) ) ;
#19360=AXIS2_PLACEMENT_3D ( 'NONE', #13576, #157, #18102 ) ;
#19365=CARTESIAN_POINT ( 'NONE',  ( 49.99999999999998579, 3.000000000000000000, 59.99999999999997868 ) ) ;
#19369=CARTESIAN_POINT ( 'NONE',  ( 50.00000000000000000, 3.000000000000000000, -60.00000000000000000 ) ) ;
#19379=EDGE_CURVE ( 'NONE', #19091, #14106, #6500, .T. ) ;
#19387=DIRECTION ( 'NONE',  ( -1.000000000000000000, 0.000000000000000000, -1.541976423090495633E-16 ) ) ;
ENDSEC;
END-ISO-10303-21;
